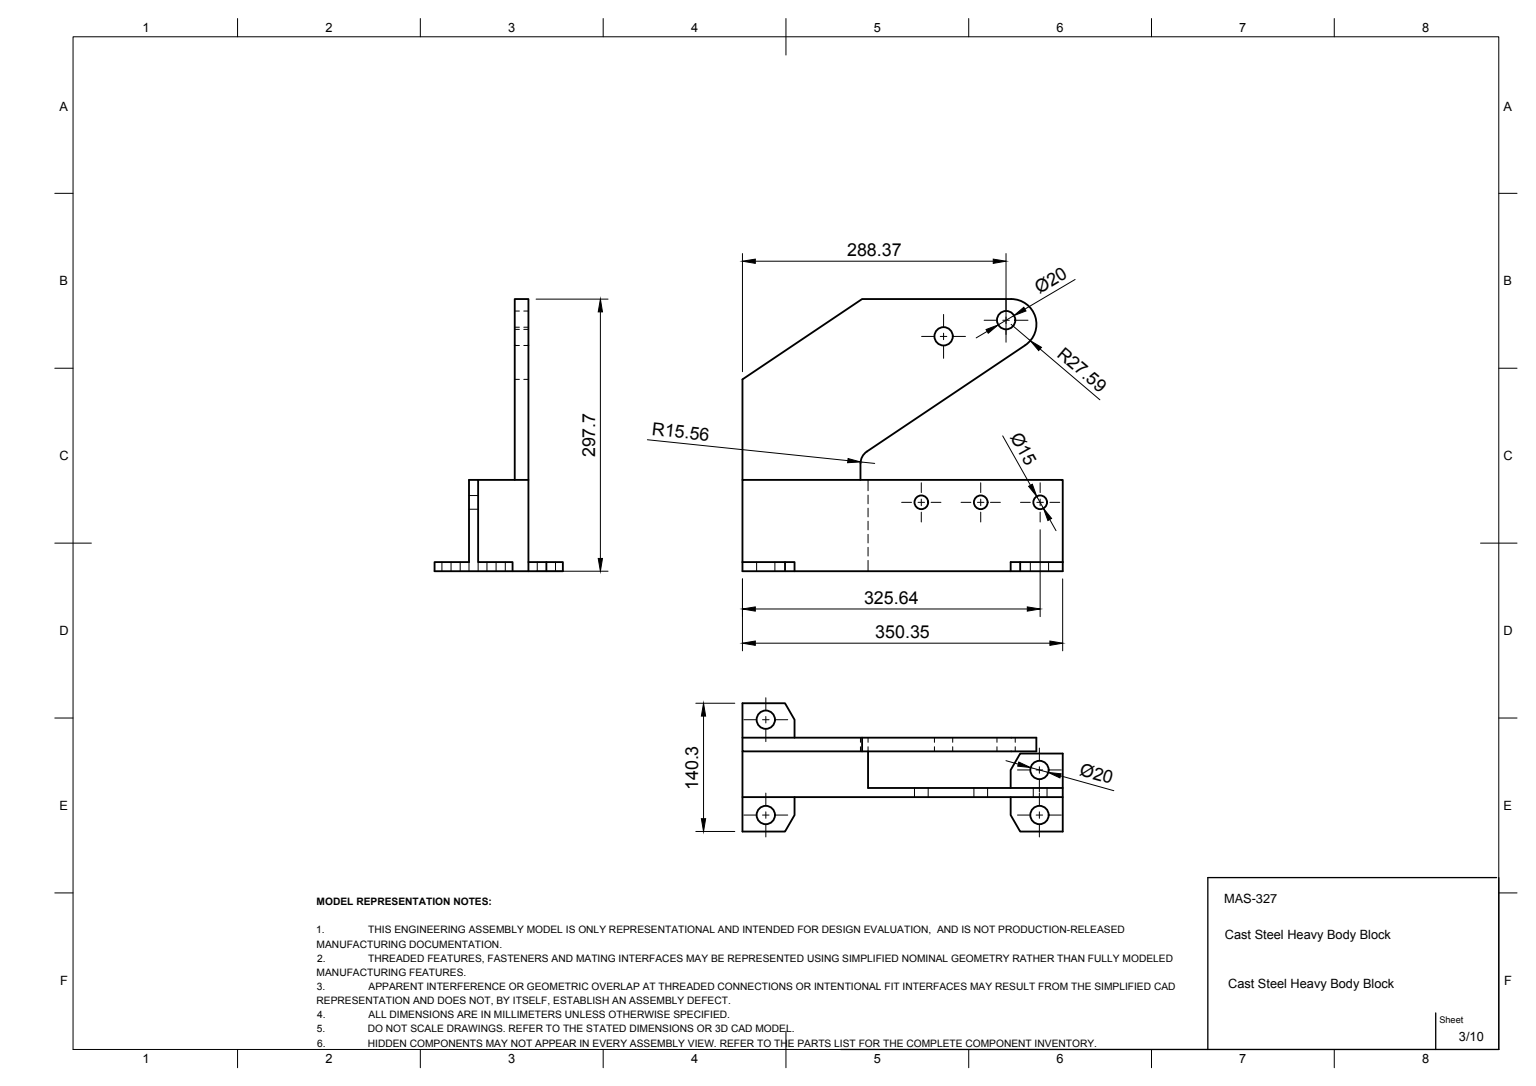
ISO-10303-21;
HEADER;
FILE_DESCRIPTION (('STEP AP214'),
    '1' );
FILE_NAME ('Cast Steel Heavy Body Block.step',
    '2026-10-06T22:16:42',
    ( '' ),
    ( '' ),
    'SwSTEP 2.0',
    'SolidWorks 2025',
    '' );
FILE_SCHEMA (( 'AUTOMOTIVE_DESIGN' ));
ENDSEC;

DATA;
#12=EDGE_LOOP ( 'NONE', ( #7089, #16124, #17025, #12845, #13237 ) ) ;
#25=CIRCLE ( 'NONE', #1445, 7.500000000000007105 ) ;
#26=EDGE_CURVE ( 'NONE', #19406, #2203, #2326, .T. ) ;
#27=ORIENTED_EDGE ( 'NONE', *, *, #7982, .F. ) ;
#40=VERTEX_POINT ( 'NONE', #786 ) ;
#42=ADVANCED_FACE ( 'NONE', ( #9065 ), #564, .F. ) ;
#49=CARTESIAN_POINT ( 'NONE',  ( -120.0322075325610598, -126.9891397928655010, -54.65701158161630246 ) ) ;
#68=VECTOR ( 'NONE', #5817, 1000.000000000000000 ) ;
#70=DIRECTION ( 'NONE',  ( -0.000000000000000000, -0.000000000000000000, 1.000000000000000000 ) ) ;
#85=VECTOR ( 'NONE', #7923, 1000.000000000000000 ) ;
#96=DIRECTION ( 'NONE',  ( -0.000000000000000000, 0.000000000000000000, 1.000000000000000000 ) ) ;
#98=FACE_OUTER_BOUND ( 'NONE', #3212, .T. ) ;
#113=ORIENTED_EDGE ( 'NONE', *, *, #2599, .F. ) ;
#114=CARTESIAN_POINT ( 'NONE',  ( -176.9699209214867324, -136.9891397928655010, -72.64809332337415526 ) ) ;
#119=VERTEX_POINT ( 'NONE', #11350 ) ;
#142=ORIENTED_EDGE ( 'NONE', *, *, #6526, .T. ) ;
#147=EDGE_LOOP ( 'NONE', ( #14360, #18336 ) ) ;
#151=DIRECTION ( 'NONE',  ( 0.000000000000000000, -1.000000000000000000, 0.000000000000000000 ) ) ;
#160=DIRECTION ( 'NONE',  ( -1.000000000000000000, 0.000000000000000000, 0.000000000000000000 ) ) ;
#167=LINE ( 'NONE', #16491, #14475 ) ;
#247=ORIENTED_EDGE ( 'NONE', *, *, #8038, .T. ) ;
#261=VECTOR ( 'NONE', #10869, 1000.000000000000000 ) ;
#269=DIRECTION ( 'NONE',  ( 0.000000000000000000, 0.000000000000000000, 1.000000000000000000 ) ) ;
#270=DIRECTION ( 'NONE',  ( -0.000000000000000000, -0.000000000000000000, -1.000000000000000000 ) ) ;
#278=ORIENTED_EDGE ( 'NONE', *, *, #11475, .T. ) ;
#284=ORIENTED_EDGE ( 'NONE', *, *, #3313, .F. ) ;
#285=VECTOR ( 'NONE', #20979, 1000.000000000000000 ) ;
#315=EDGE_CURVE ( 'NONE', #5215, #4975, #25, .T. ) ;
#328=FACE_OUTER_BOUND ( 'NONE', #18449, .T. ) ;
#380=FACE_OUTER_BOUND ( 'NONE', #4715, .T. ) ;
#417=VERTEX_POINT ( 'NONE', #9257 ) ;
#418=CIRCLE ( 'NONE', #12730, 27.58651506682278765 ) ;
#431=DIRECTION ( 'NONE',  ( 0.000000000000000000, 0.000000000000000000, 1.000000000000000000 ) ) ;
#437=PLANE ( 'NONE',  #12824 ) ;
#465=PLANE ( 'NONE',  #7815 ) ;
#468=ORIENTED_EDGE ( 'NONE', *, *, #12037, .F. ) ;
#478=FACE_OUTER_BOUND ( 'NONE', #9416, .T. ) ;
#509=VECTOR ( 'NONE', #17176, 1000.000000000000000 ) ;
#516=ADVANCED_FACE ( 'NONE', ( #17287, #19278 ), #15850, .F. ) ;
#522=ORIENTED_EDGE ( 'NONE', *, *, #11916, .F. ) ;
#541=CIRCLE ( 'NONE', #5131, 10.00000000000000888 ) ;
#559=FACE_OUTER_BOUND ( 'NONE', #21629, .T. ) ;
#564=CYLINDRICAL_SURFACE ( 'NONE', #18674, 10.00000000000000888 ) ;
#566=ADVANCED_FACE ( 'NONE', ( #7498 ), #12330, .F. ) ;
#590=AXIS2_PLACEMENT_3D ( 'NONE', #17670, #14043, #3917 ) ;
#593=EDGE_CURVE ( 'NONE', #21705, #4967, #4602, .T. ) ;
#601=EDGE_CURVE ( 'NONE', #16938, #20322, #15854, .T. ) ;
#609=LINE ( 'NONE', #7345, #1308 ) ;
#633=CIRCLE ( 'NONE', #13999, 7.500000000000000000 ) ;
#657=DIRECTION ( 'NONE',  ( 0.000000000000000000, 0.000000000000000000, 1.000000000000000000 ) ) ;
#658=ORIENTED_EDGE ( 'NONE', *, *, #12587, .F. ) ;
#668=AXIS2_PLACEMENT_3D ( 'NONE', #14423, #4498, #6045 ) ;
#677=ADVANCED_FACE ( 'NONE', ( #16611 ), #4491, .T. ) ;
#678=CARTESIAN_POINT ( 'NONE',  ( 147.8787791192428074, -126.9891397928655010, 49.65701158161629536 ) ) ;
#682=ORIENTED_EDGE ( 'NONE', *, *, #18825, .F. ) ;
#684=VECTOR ( 'NONE', #722, 1000.000000000000000 ) ;
#706=VERTEX_POINT ( 'NONE', #21264 ) ;
#722=DIRECTION ( 'NONE',  ( 0.000000000000000000, 0.000000000000000000, 1.000000000000000000 ) ) ;
#724=CYLINDRICAL_SURFACE ( 'NONE', #15405, 7.500000000000007105 ) ;
#735=VERTEX_POINT ( 'NONE', #15411 ) ;
#736=VECTOR ( 'NONE', #19488, 1000.000000000000000 ) ;
#761=CARTESIAN_POINT ( 'NONE',  ( 0.000000000000000000, -126.9891397928655010, 0.000000000000000000 ) ) ;
#766=ORIENTED_EDGE ( 'NONE', *, *, #1366, .T. ) ;
#779=DIRECTION ( 'NONE',  ( 0.000000000000000000, 0.000000000000000000, 1.000000000000000000 ) ) ;
#784=VERTEX_POINT ( 'NONE', #6929 ) ;
#786=CARTESIAN_POINT ( 'NONE',  ( -130.4480969619998234, -126.9891397928655010, 67.64809332337415526 ) ) ;
#803=DIRECTION ( 'NONE',  ( 0.000000000000000000, 0.000000000000000000, 1.000000000000000000 ) ) ;
#805=LINE ( 'NONE', #10631, #5353 ) ;
#818=ORIENTED_EDGE ( 'NONE', *, *, #4976, .F. ) ;
#847=ORIENTED_EDGE ( 'NONE', *, *, #6809, .F. ) ;
#850=AXIS2_PLACEMENT_3D ( 'NONE', #17976, #8078, #1233 ) ;
#858=DIRECTION ( 'NONE',  ( 1.000000000000000000, 0.000000000000000000, 5.966140889015784385E-16 ) ) ;
#863=( NAMED_UNIT ( * ) SI_UNIT ( $, .STERADIAN. ) SOLID_ANGLE_UNIT ( ) );
#879=LINE ( 'NONE', #9488, #12922 ) ;
#929=EDGE_CURVE ( 'NONE', #15878, #9201, #3287, .T. ) ;
#943=CYLINDRICAL_SURFACE ( 'NONE', #4707, 10.00000000000000888 ) ;
#965=DIRECTION ( 'NONE',  ( 0.000000000000000000, -1.000000000000000000, 0.000000000000000000 ) ) ;
#970=FILL_AREA_STYLE ('',( #2836 ) ) ;
#1005=DIRECTION ( 'NONE',  ( 0.000000000000000000, 0.000000000000000000, -1.000000000000000000 ) ) ;
#1023=CARTESIAN_POINT ( 'NONE',  ( 116.9721770337685740, 133.1239846058259388, -19.99999999999999289 ) ) ;
#1032=AXIS2_PLACEMENT_3D ( 'NONE', #6238, #19694, #16478 ) ;
#1085=CARTESIAN_POINT ( 'NONE',  ( -120.0322075325610598, -126.9891397928655010, -54.65701158161630246 ) ) ;
#1093=ORIENTED_EDGE ( 'NONE', *, *, #6809, .T. ) ;
#1101=LINE ( 'NONE', #19613, #20236 ) ;
#1116=VERTEX_POINT ( 'NONE', #18932 ) ;
#1131=CARTESIAN_POINT ( 'NONE',  ( -176.9699209214867608, -126.9891397928655010, -35.00000000000000000 ) ) ;
#1139=DIRECTION ( 'NONE',  ( -1.233581138472395521E-15, -0.000000000000000000, 1.000000000000000000 ) ) ;
#1143=ORIENTED_EDGE ( 'NONE', *, *, #9526, .F. ) ;
#1149=DIRECTION ( 'NONE',  ( 0.5010362705417042983, 0.000000000000000000, 0.8654262854811264338 ) ) ;
#1171=ORIENTED_EDGE ( 'NONE', *, *, #13365, .T. ) ;
#1192=DIRECTION ( 'NONE',  ( 1.000000000000000000, 0.000000000000000000, 0.000000000000000000 ) ) ;
#1194=DIRECTION ( 'NONE',  ( 1.000000000000000000, 0.000000000000000000, 0.000000000000000000 ) ) ;
#1208=CARTESIAN_POINT ( 'NONE',  ( -176.9699209214867892, 72.84679049016736485, -25.00000000000000000 ) ) ;
#1224=ORIENTED_EDGE ( 'NONE', *, *, #1690, .F. ) ;
#1225=ORIENTED_EDGE ( 'NONE', *, *, #2133, .T. ) ;
#1233=DIRECTION ( 'NONE',  ( 1.000000000000000000, 0.000000000000000000, 0.000000000000000000 ) ) ;
#1237=CARTESIAN_POINT ( 'NONE',  ( 148.6725454929228079, -61.68114226949890622, 19.99999999999998934 ) ) ;
#1279=ORIENTED_EDGE ( 'NONE', *, *, #10623, .F. ) ;
#1280=ORIENTED_EDGE ( 'NONE', *, *, #9639, .T. ) ;
#1282=EDGE_CURVE ( 'NONE', #4009, #10043, #14611, .T. ) ;
#1302=DIRECTION ( 'NONE',  ( 0.000000000000000000, -1.000000000000000000, 0.000000000000000000 ) ) ;
#1304=CARTESIAN_POINT ( 'NONE',  ( 43.01140435219951996, 119.9070776186055838, -35.00000000000000000 ) ) ;
#1308=VECTOR ( 'NONE', #20782, 1000.000000000000000 ) ;
#1344=DIRECTION ( 'NONE',  ( -0.000000000000000000, 1.000000000000000000, 0.000000000000000000 ) ) ;
#1366=EDGE_CURVE ( 'NONE', #10070, #12769, #541, .T. ) ;
#1408=DIRECTION ( 'NONE',  ( 0.000000000000000000, -1.000000000000000000, 0.000000000000000000 ) ) ;
#1445=AXIS2_PLACEMENT_3D ( 'NONE', #7171, #18740, #10262 ) ;
#1463=ORIENTED_EDGE ( 'NONE', *, *, #1366, .F. ) ;
#1497=CARTESIAN_POINT ( 'NONE',  ( 126.8576204525573274, -136.9891397928655010, 67.64809332337412684 ) ) ;
#1507=FACE_OUTER_BOUND ( 'NONE', #6778, .T. ) ;
#1510=CARTESIAN_POINT ( 'NONE',  ( 116.9721770337685740, 133.1239846058259388, -35.00000000000000000 ) ) ;
#1512=DIRECTION ( 'NONE',  ( 0.000000000000000000, -1.000000000000000000, 0.000000000000000000 ) ) ;
#1527=ORIENTED_EDGE ( 'NONE', *, *, #18029, .T. ) ;
#1535=CARTESIAN_POINT ( 'NONE',  ( -120.0322075325610740, -126.9891397928655010, 49.65701158161630957 ) ) ;
#1538=ADVANCED_FACE ( 'NONE', ( #15287 ), #10546, .F. ) ;
#1542=CARTESIAN_POINT ( 'NONE',  ( -151.4692556286852891, -126.9891397928655010, -64.65701158161634510 ) ) ;
#1543=EDGE_CURVE ( 'NONE', #18069, #12813, #20253, .T. ) ;
#1569=DIRECTION ( 'NONE',  ( -1.000000000000000000, 0.000000000000000000, 0.000000000000000000 ) ) ;
#1573=VERTEX_POINT ( 'NONE', #18482 ) ;
#1581=AXIS2_PLACEMENT_3D ( 'NONE', #1237, #19759, #16328 ) ;
#1601=AXIS2_PLACEMENT_3D ( 'NONE', #19582, #1512, #8350 ) ;
#1608=VERTEX_POINT ( 'NONE', #16926 ) ;
#1612=CYLINDRICAL_SURFACE ( 'NONE', #21460, 7.500000000000007105 ) ;
#1631=DIRECTION ( 'NONE',  ( 0.000000000000000000, -1.000000000000000000, 0.000000000000000000 ) ) ;
#1635=DIRECTION ( 'NONE',  ( 1.000000000000000000, 0.000000000000000000, 0.000000000000000000 ) ) ;
#1636=EDGE_LOOP ( 'NONE', ( #13666, #2702 ) ) ;
#1646=LINE ( 'NONE', #11664, #7653 ) ;
#1662=EDGE_CURVE ( 'NONE', #9722, #11465, #14251, .T. ) ;
#1665=EDGE_LOOP ( 'NONE', ( #5611, #19532, #4554, #12412 ) ) ;
#1668=EDGE_CURVE ( 'NONE', #4967, #19403, #16139, .T. ) ;
#1680=CARTESIAN_POINT ( 'NONE',  ( 18.67254549292281141, -61.68114226949890622, 30.00000000000000000 ) ) ;
#1690=EDGE_CURVE ( 'NONE', #12769, #10070, #4754, .T. ) ;
#1692=CARTESIAN_POINT ( 'NONE',  ( -39.63192160874135084, -37.13255853780189852, 20.00000000000002132 ) ) ;
#1696=VERTEX_POINT ( 'NONE', #5891 ) ;
#1702=DIRECTION ( 'NONE',  ( 0.000000000000000000, -1.000000000000000000, 0.000000000000000000 ) ) ;
#1707=DIRECTION ( 'NONE',  ( 0.000000000000000000, -1.000000000000000000, 0.000000000000000000 ) ) ;
#1709=CARTESIAN_POINT ( 'NONE',  ( -151.4692556286852891, -136.9891397928655010, 39.65701158161630246 ) ) ;
#1729=CARTESIAN_POINT ( 'NONE',  ( 173.3794444120442506, -126.9891397928655010, 67.64809332337412684 ) ) ;
#1741=DIRECTION ( 'NONE',  ( -0.000000000000000000, -0.000000000000000000, 1.000000000000000000 ) ) ;
#1760=CARTESIAN_POINT ( 'NONE',  ( -176.9699209214867608, -136.9891397928655010, -35.00000000000000000 ) ) ;
#1768=DIRECTION ( 'NONE',  ( 1.000000000000000000, 0.000000000000000000, 5.966140889015784385E-16 ) ) ;
#1773=EDGE_CURVE ( 'NONE', #11679, #1573, #7680, .T. ) ;
#1794=AXIS2_PLACEMENT_3D ( 'NONE', #761, #5605, #2201 ) ;
#1804=ORIENTED_EDGE ( 'NONE', *, *, #20245, .T. ) ;
#1807=ORIENTED_EDGE ( 'NONE', *, *, #15853, .T. ) ;
#1836=VECTOR ( 'NONE', #5777, 1000.000000000000000 ) ;
#1840=CARTESIAN_POINT ( 'NONE',  ( 26.17254549292281141, -61.68114226949890622, 30.00000000000000000 ) ) ;
#1856=CARTESIAN_POINT ( 'NONE',  ( 116.9721770337685740, 133.1239846058259388, -19.99999999999999289 ) ) ;
#1866=CARTESIAN_POINT ( 'NONE',  ( -40.97538603781489996, -6.141859983696325465, -25.00000000000000000 ) ) ;
#1898=AXIS2_PLACEMENT_3D ( 'NONE', #17581, #5791, #9447 ) ;
#1899=ORIENTED_EDGE ( 'NONE', *, *, #8843, .F. ) ;
#1913=CYLINDRICAL_SURFACE ( 'NONE', #20496, 10.00000000000003730 ) ;
#1934=EDGE_CURVE ( 'NONE', #21705, #12683, #2918, .T. ) ;
#1936=EDGE_LOOP ( 'NONE', ( #10832, #15493, #3293, #10748, #3973, #12663, #1527, #9500 ) ) ;
#1979=VECTOR ( 'NONE', #8089, 1000.000000000000000 ) ;
#1997=VECTOR ( 'NONE', #12476, 1000.000000000000000 ) ;
#2032=CYLINDRICAL_SURFACE ( 'NONE', #3445, 27.58651506682278765 ) ;
#2041=CARTESIAN_POINT ( 'NONE',  ( 126.8576204525573274, -136.9891397928655010, -17.64809332337413750 ) ) ;
#2042=CARTESIAN_POINT ( 'NONE',  ( -88.69383338279318707, 132.1114735047150646, -19.99999999999996803 ) ) ;
#2046=AXIS2_PLACEMENT_3D ( 'NONE', #16795, #15260, #13597 ) ;
#2082=DIRECTION ( 'NONE',  ( -1.000000000000000000, 0.000000000000000000, -0.000000000000000000 ) ) ;
#2089=DIRECTION ( 'NONE',  ( 1.186952418100008983E-16, 0.000000000000000000, 1.000000000000000000 ) ) ;
#2092=CARTESIAN_POINT ( 'NONE',  ( 173.3794444120442222, -354.7018910364275257, 19.99999999999999645 ) ) ;
#2095=EDGE_LOOP ( 'NONE', ( #16991, #14494, #15108, #12297 ) ) ;
#2133=EDGE_CURVE ( 'NONE', #3147, #7116, #5434, .T. ) ;
#2143=DIRECTION ( 'NONE',  ( 0.000000000000000000, -1.000000000000000000, 0.000000000000000000 ) ) ;
#2145=ORIENTED_EDGE ( 'NONE', *, *, #9831, .T. ) ;
#2157=CARTESIAN_POINT ( 'NONE',  ( 26.17254549292281141, -61.68114226949890622, -46.21320343559645494 ) ) ;
#2160=CARTESIAN_POINT ( 'NONE',  ( 101.4021762516569822, 137.5714195593754710, -35.00000000000000000 ) ) ;
#2161=CARTESIAN_POINT ( 'NONE',  ( 53.01140435219953417, 119.9070776186055838, -35.00000000000000000 ) ) ;
#2175=ORIENTED_EDGE ( 'NONE', *, *, #7095, .T. ) ;
#2177=CARTESIAN_POINT ( 'NONE',  ( -151.4692556286852891, -126.9891397928655010, 39.65701158161630246 ) ) ;
#2188=AXIS2_PLACEMENT_3D ( 'NONE', #13387, #4899, #6555 ) ;
#2201=DIRECTION ( 'NONE',  ( 0.000000000000000000, -0.000000000000000000, -1.000000000000000000 ) ) ;
#2203=VERTEX_POINT ( 'NONE', #3476 ) ;
#2258=CARTESIAN_POINT ( 'NONE',  ( -151.4692556286852891, -136.9891397928655010, 59.65701158161632378 ) ) ;
#2276=EDGE_CURVE ( 'NONE', #17291, #7232, #14977, .T. ) ;
#2280=DIRECTION ( 'NONE',  ( 1.000000000000000000, 0.000000000000000000, 0.000000000000000000 ) ) ;
#2294=CARTESIAN_POINT ( 'NONE',  ( 144.5586921005913439, 482.8605407899846682, -19.99999999999999645 ) ) ;
#2326=LINE ( 'NONE', #2647, #3184 ) ;
#2328=ADVANCED_FACE ( 'NONE', ( #4870, #11807 ), #14783, .T. ) ;
#2331=ORIENTED_EDGE ( 'NONE', *, *, #10158, .F. ) ;
#2334=CIRCLE ( 'NONE', #19236, 10.00000000000003730 ) ;
#2344=VECTOR ( 'NONE', #431, 1000.000000000000000 ) ;
#2377=ADVANCED_FACE ( 'NONE', ( #13468 ), #13138, .F. ) ;
#2403=CARTESIAN_POINT ( 'NONE',  ( 0.000000000000000000, 0.000000000000000000, 0.000000000000000000 ) ) ;
#2404=DIRECTION ( 'NONE',  ( -0.000000000000000000, -0.000000000000000000, 1.000000000000000000 ) ) ;
#2405=DIRECTION ( 'NONE',  ( 0.000000000000000000, 0.000000000000000000, -1.000000000000000000 ) ) ;
#2456=ORIENTED_EDGE ( 'NONE', *, *, #8916, .F. ) ;
#2466=ORIENTED_EDGE ( 'NONE', *, *, #13663, .T. ) ;
#2479=DIRECTION ( 'NONE',  ( -0.000000000000000000, -0.000000000000000000, 1.000000000000000000 ) ) ;
#2496=DIRECTION ( 'NONE',  ( -0.000000000000000000, -0.000000000000000000, 1.000000000000000000 ) ) ;
#2507=LINE ( 'NONE', #19268, #16704 ) ;
#2512=SURFACE_STYLE_FILL_AREA ( #970 ) ;
#2527=AXIS2_PLACEMENT_3D ( 'NONE', #10957, #17666, #9308 ) ;
#2536=CARTESIAN_POINT ( 'NONE',  ( -176.9699209214867892, 72.84679049016739327, -19.99999999999995737 ) ) ;
#2549=EDGE_CURVE ( 'NONE', #15790, #784, #8294, .T. ) ;
#2562=DIRECTION ( 'NONE',  ( -0.000000000000000000, -0.000000000000000000, -1.000000000000000000 ) ) ;
#2563=EDGE_LOOP ( 'NONE', ( #11816, #5747, #14579, #3772 ) ) ;
#2574=VERTEX_POINT ( 'NONE', #13676 ) ;
#2580=CARTESIAN_POINT ( 'NONE',  ( 173.3794444120442506, -136.9891397928655010, -17.64809332337413750 ) ) ;
#2599=EDGE_CURVE ( 'NONE', #3989, #14342, #7299, .T. ) ;
#2611=DIRECTION ( 'NONE',  ( 1.000000000000000000, 0.000000000000000000, 0.000000000000000000 ) ) ;
#2616=SURFACE_SIDE_STYLE ('',( #2512 ) ) ;
#2625=DIRECTION ( 'NONE',  ( 0.000000000000000000, -1.000000000000000000, 0.000000000000000000 ) ) ;
#2637=LINE ( 'NONE', #1208, #3416 ) ;
#2639=DIRECTION ( 'NONE',  ( 0.000000000000000000, 0.000000000000000000, -1.000000000000000000 ) ) ;
#2647=CARTESIAN_POINT ( 'NONE',  ( 144.5586921005913439, 133.1239846058259388, -25.00000000000000000 ) ) ;
#2663=UNCERTAINTY_MEASURE_WITH_UNIT (LENGTH_MEASURE( 1.000000000000000082E-05 ), #12101, 'distance_accuracy_value', 'NONE');
#2673=EDGE_LOOP ( 'NONE', ( #7016, #20805 ) ) ;
#2675=CIRCLE ( 'NONE', #7981, 10.00000000000000888 ) ;
#2702=ORIENTED_EDGE ( 'NONE', *, *, #5054, .F. ) ;
#2719=CARTESIAN_POINT ( 'NONE',  ( 116.9721770337685882, 160.7104996726487514, -35.00000000000000000 ) ) ;
#2737=CARTESIAN_POINT ( 'NONE',  ( -47.86331837773882825, -37.13255853780189852, -25.00000000000000000 ) ) ;
#2740=VECTOR ( 'NONE', #14647, 1000.000000000000000 ) ;
#2742=VERTEX_POINT ( 'NONE', #3765 ) ;
#2748=CARTESIAN_POINT ( 'NONE',  ( 26.17254549292281141, -61.68114226949890622, 20.00000000000000355 ) ) ;
#2774=ADVANCED_FACE ( 'NONE', ( #4505 ), #14211, .F. ) ;
#2782=ORIENTED_EDGE ( 'NONE', *, *, #11167, .F. ) ;
#2798=EDGE_CURVE ( 'NONE', #12363, #19770, #19292, .T. ) ;
#2800=VECTOR ( 'NONE', #6103, 1000.000000000000000 ) ;
#2814=LINE ( 'NONE', #14493, #10358 ) ;
#2836=FILL_AREA_STYLE_COLOUR ( '', #20940 ) ;
#2837=CARTESIAN_POINT ( 'NONE',  ( -120.0322075325610740, -126.9891397928655010, 49.65701158161630957 ) ) ;
#2838=CARTESIAN_POINT ( 'NONE',  ( 173.3794444120442506, -126.9891397928655010, 19.99999999999999645 ) ) ;
#2839=LINE ( 'NONE', #9580, #85 ) ;
#2841=CARTESIAN_POINT ( 'NONE',  ( 116.9721770337685740, 133.1239846058259388, -25.00000000000000000 ) ) ;
#2853=DIRECTION ( 'NONE',  ( -0.000000000000000000, -0.000000000000000000, 1.000000000000000000 ) ) ;
#2856=DIRECTION ( 'NONE',  ( 1.000000000000000000, -0.000000000000000000, -0.000000000000000000 ) ) ;
#2872=ORIENTED_EDGE ( 'NONE', *, *, #5164, .F. ) ;
#2873=ORIENTED_EDGE ( 'NONE', *, *, #19692, .F. ) ;
#2880=CIRCLE ( 'NONE', #15211, 10.00000000000000888 ) ;
#2918=LINE ( 'NONE', #6560, #10778 ) ;
#2932=EDGE_LOOP ( 'NONE', ( #3098, #5240 ) ) ;
#2954=LINE ( 'NONE', #10911, #8544 ) ;
#2957=DIRECTION ( 'NONE',  ( 0.000000000000000000, -1.000000000000000000, 0.000000000000000000 ) ) ;
#2958=ADVANCED_FACE ( 'NONE', ( #16298 ), #19724, .T. ) ;
#2967=ADVANCED_BREP_SHAPE_REPRESENTATION ( '', ( #7648, #12657 ), #7388 ) ;
#2984=ORIENTED_EDGE ( 'NONE', *, *, #11356, .F. ) ;
#2994=VECTOR ( 'NONE', #5145, 1000.000000000000000 ) ;
#3009=ORIENTED_EDGE ( 'NONE', *, *, #8423, .F. ) ;
#3014=AXIS2_PLACEMENT_3D ( 'NONE', #17733, #19730, #2639 ) ;
#3015=EDGE_LOOP ( 'NONE', ( #12043, #12503, #17690, #7873 ) ) ;
#3022=CARTESIAN_POINT ( 'NONE',  ( -176.9699209214867892, -37.13255853780189852, 30.00000000000000000 ) ) ;
#3035=ORIENTED_EDGE ( 'NONE', *, *, #11167, .T. ) ;
#3041=EDGE_LOOP ( 'NONE', ( #18081, #20830, #4851, #15021 ) ) ;
#3043=AXIS2_PLACEMENT_3D ( 'NONE', #14344, #7530, #10618 ) ;
#3059=FACE_OUTER_BOUND ( 'NONE', #1936, .T. ) ;
#3079=DIRECTION ( 'NONE',  ( 5.966140889015784385E-16, 0.000000000000000000, -1.000000000000000000 ) ) ;
#3081=CARTESIAN_POINT ( 'NONE',  ( 11.17254549292281318, -61.68114226949890622, 20.00000000000000355 ) ) ;
#3084=CARTESIAN_POINT ( 'NONE',  ( 83.67254549292280785, -61.68114226949890622, 20.00000000000000355 ) ) ;
#3098=ORIENTED_EDGE ( 'NONE', *, *, #12468, .F. ) ;
#3099=ORIENTED_EDGE ( 'NONE', *, *, #7039, .F. ) ;
#3110=DIRECTION ( 'NONE',  ( 0.000000000000000000, -1.000000000000000000, 0.000000000000000000 ) ) ;
#3113=CARTESIAN_POINT ( 'NONE',  ( 141.1725454929228079, -61.68114226949890622, 30.00000000000000000 ) ) ;
#3147=VERTEX_POINT ( 'NONE', #19051 ) ;
#3159=EDGE_CURVE ( 'NONE', #2574, #14607, #20383, .T. ) ;
#3179=ORIENTED_EDGE ( 'NONE', *, *, #26, .F. ) ;
#3183=CARTESIAN_POINT ( 'NONE',  ( 147.8787791192428074, -136.9891397928655010, 10.34298841838370642 ) ) ;
#3184=VECTOR ( 'NONE', #9389, 1000.000000000000000 ) ;
#3193=FACE_OUTER_BOUND ( 'NONE', #7898, .T. ) ;
#3212=EDGE_LOOP ( 'NONE', ( #10152, #12911, #16288, #16341 ) ) ;
#3240=ORIENTED_EDGE ( 'NONE', *, *, #16105, .T. ) ;
#3275=DIRECTION ( 'NONE',  ( -1.000000000000000000, 0.000000000000000000, -2.437363037925170562E-16 ) ) ;
#3276=EDGE_CURVE ( 'NONE', #8458, #14342, #14465, .T. ) ;
#3280=LINE ( 'NONE', #12898, #5354 ) ;
#3282=CARTESIAN_POINT ( 'NONE',  ( 0.000000000000000000, -37.13255853780189852, 30.00000000000000000 ) ) ;
#3287=LINE ( 'NONE', #16720, #10407 ) ;
#3291=CIRCLE ( 'NONE', #15601, 10.00000000000003730 ) ;
#3293=ORIENTED_EDGE ( 'NONE', *, *, #3630, .T. ) ;
#3313=EDGE_CURVE ( 'NONE', #15277, #4525, #17769, .T. ) ;
#3321=ORIENTED_EDGE ( 'NONE', *, *, #8843, .T. ) ;
#3323=ORIENTED_EDGE ( 'NONE', *, *, #1773, .F. ) ;
#3329=CARTESIAN_POINT ( 'NONE',  ( 0.000000000000000000, -126.9891397928655010, 0.000000000000000000 ) ) ;
#3332=FACE_OUTER_BOUND ( 'NONE', #19635, .T. ) ;
#3337=ORIENTED_EDGE ( 'NONE', *, *, #6526, .F. ) ;
#3353=CARTESIAN_POINT ( 'NONE',  ( -151.4692556286852891, -136.9891397928655010, -54.65701158161630246 ) ) ;
#3363=DIRECTION ( 'NONE',  ( 1.000000000000000000, 0.000000000000000000, 0.000000000000000000 ) ) ;
#3378=ORIENTED_EDGE ( 'NONE', *, *, #4559, .T. ) ;
#3391=EDGE_CURVE ( 'NONE', #13430, #16995, #21315, .T. ) ;
#3396=DIRECTION ( 'NONE',  ( -0.5010362705417047424, 0.000000000000000000, -0.8654262854811261008 ) ) ;
#3408=EDGE_LOOP ( 'NONE', ( #14606, #4517, #12471, #2782 ) ) ;
#3416=VECTOR ( 'NONE', #779, 1000.000000000000000 ) ;
#3436=VECTOR ( 'NONE', #13943, 1000.000000000000000 ) ;
#3445=AXIS2_PLACEMENT_3D ( 'NONE', #18461, #269, #3363 ) ;
#3476=CARTESIAN_POINT ( 'NONE',  ( 144.5586921005913439, 133.1239846058259388, -19.99999999999999645 ) ) ;
#3485=ORIENTED_EDGE ( 'NONE', *, *, #21498, .T. ) ;
#3495=FACE_OUTER_BOUND ( 'NONE', #12, .T. ) ;
#3508=CARTESIAN_POINT ( 'NONE',  ( 147.8787791192428074, -126.9891397928655010, 10.34298841838370642 ) ) ;
#3564=EDGE_CURVE ( 'NONE', #1573, #10861, #4803, .T. ) ;
#3569=ORIENTED_EDGE ( 'NONE', *, *, #6191, .F. ) ;
#3577=FACE_OUTER_BOUND ( 'NONE', #19092, .T. ) ;
#3598=CIRCLE ( 'NONE', #12744, 10.00000000000003730 ) ;
#3630=EDGE_CURVE ( 'NONE', #12363, #20108, #7922, .T. ) ;
#3648=FACE_OUTER_BOUND ( 'NONE', #12386, .T. ) ;
#3667=EDGE_LOOP ( 'NONE', ( #7526, #9262, #18046, #20185, #3337, #5414, #10888, #19284, #4437, #9397, #14577, #6175, #1280 ) ) ;
#3674=ORIENTED_EDGE ( 'NONE', *, *, #13573, .T. ) ;
#3677=CARTESIAN_POINT ( 'NONE',  ( -151.4692556286852891, -136.9891397928655010, -64.65701158161634510 ) ) ;
#3684=EDGE_CURVE ( 'NONE', #9201, #4525, #14843, .T. ) ;
#3687=FACE_OUTER_BOUND ( 'NONE', #19743, .T. ) ;
#3730=DIRECTION ( 'NONE',  ( 1.000000000000000000, 0.000000000000000000, -1.257660470541341077E-16 ) ) ;
#3755=DIRECTION ( 'NONE',  ( 1.000000000000000000, 0.000000000000000000, -0.000000000000000000 ) ) ;
#3758=AXIS2_PLACEMENT_3D ( 'NONE', #6028, #965, #2405 ) ;
#3765=CARTESIAN_POINT ( 'NONE',  ( 91.17254549292282206, -61.68114226949890622, 20.00000000000000355 ) ) ;
#3772=ORIENTED_EDGE ( 'NONE', *, *, #2599, .T. ) ;
#3786=CARTESIAN_POINT ( 'NONE',  ( 126.8576204525573274, -126.9891397928655010, -17.64809332337413750 ) ) ;
#3789=AXIS2_PLACEMENT_3D ( 'NONE', #3084, #18514, #10036 ) ;
#3796=CARTESIAN_POINT ( 'NONE',  ( 156.1725454929228079, -61.68114226949890622, 30.00000000000000000 ) ) ;
#3805=VECTOR ( 'NONE', #20027, 1000.000000000000000 ) ;
#3833=ADVANCED_FACE ( 'NONE', ( #16828 ), #15183, .F. ) ;
#3873=DIRECTION ( 'NONE',  ( -0.000000000000000000, -0.000000000000000000, -1.000000000000000000 ) ) ;
#3883=ORIENTED_EDGE ( 'NONE', *, *, #18144, .F. ) ;
#3903=ADVANCED_FACE ( 'NONE', ( #13739 ), #8684, .T. ) ;
#3917=DIRECTION ( 'NONE',  ( 0.000000000000000000, 0.000000000000000000, -1.000000000000000000 ) ) ;
#3920=CARTESIAN_POINT ( 'NONE',  ( 18.67254549292281141, -61.68114226949890622, -46.21320343559645494 ) ) ;
#3953=( NAMED_UNIT ( * ) PLANE_ANGLE_UNIT ( ) SI_UNIT ( $, .RADIAN. ) );
#3973=ORIENTED_EDGE ( 'NONE', *, *, #14257, .F. ) ;
#3983=DIRECTION ( 'NONE',  ( 0.000000000000000000, 0.000000000000000000, 1.000000000000000000 ) ) ;
#3989=VERTEX_POINT ( 'NONE', #11873 ) ;
#4009=VERTEX_POINT ( 'NONE', #3508 ) ;
#4021=CARTESIAN_POINT ( 'NONE',  ( 126.8576204525573274, -136.9891397928655010, 67.64809332337412684 ) ) ;
#4026=DIRECTION ( 'NONE',  ( 0.000000000000000000, 0.000000000000000000, -1.000000000000000000 ) ) ;
#4035=LINE ( 'NONE', #17574, #9321 ) ;
#4051=DIRECTION ( 'NONE',  ( 0.8302490056034136368, 0.5573926701119623628, 0.000000000000000000 ) ) ;
#4082=LINE ( 'NONE', #16079, #10825 ) ;
#4084=CARTESIAN_POINT ( 'NONE',  ( 116.4417310231185780, -136.9891397928655010, 30.00000000000000000 ) ) ;
#4086=CARTESIAN_POINT ( 'NONE',  ( 147.8787791192428074, -126.9891397928655010, -9.657011581616311346 ) ) ;
#4091=ORIENTED_EDGE ( 'NONE', *, *, #9801, .T. ) ;
#4104=LINE ( 'NONE', #12590, #16410 ) ;
#4110=AXIS2_PLACEMENT_3D ( 'NONE', #21112, #19234, #13938 ) ;
#4113=DIRECTION ( 'NONE',  ( 0.000000000000000000, -1.000000000000000000, 0.000000000000000000 ) ) ;
#4134=DIRECTION ( 'NONE',  ( 0.000000000000000000, 0.000000000000000000, 1.000000000000000000 ) ) ;
#4138=CARTESIAN_POINT ( 'NONE',  ( -176.9699209214867608, -126.9891397928655010, -35.00000000000000000 ) ) ;
#4145=CARTESIAN_POINT ( 'NONE',  ( 116.4417310231185780, -126.9891397928655010, 49.65701158161629536 ) ) ;
#4198=DIRECTION ( 'NONE',  ( -0.000000000000000000, -0.000000000000000000, 1.000000000000000000 ) ) ;
#4199=ORIENTED_EDGE ( 'NONE', *, *, #8423, .T. ) ;
#4205=ORIENTED_EDGE ( 'NONE', *, *, #14991, .T. ) ;
#4218=DIRECTION ( 'NONE',  ( 0.000000000000000000, -1.000000000000000000, 0.000000000000000000 ) ) ;
#4238=DIRECTION ( 'NONE',  ( -1.000000000000000000, -0.000000000000000000, -0.000000000000000000 ) ) ;
#4244=EDGE_CURVE ( 'NONE', #14342, #3147, #17903, .T. ) ;
#4268=FACE_OUTER_BOUND ( 'NONE', #3015, .T. ) ;
#4279=LINE ( 'NONE', #4605, #7485 ) ;
#4283=ADVANCED_FACE ( 'NONE', ( #16257, #8227, #6228, #19564 ), #18247, .F. ) ;
#4286=AXIS2_PLACEMENT_3D ( 'NONE', #11428, #15955, #4377 ) ;
#4299=ORIENTED_EDGE ( 'NONE', *, *, #12587, .T. ) ;
#4318=CARTESIAN_POINT ( 'NONE',  ( -120.0322075325610740, -126.9891397928655010, 49.65701158161630957 ) ) ;
#4320=CARTESIAN_POINT ( 'NONE',  ( 173.3794444120442506, -126.9891397928655010, -17.64809332337413750 ) ) ;
#4343=DIRECTION ( 'NONE',  ( -1.140132994654635861E-16, -0.000000000000000000, -1.000000000000000000 ) ) ;
#4357=ORIENTED_EDGE ( 'NONE', *, *, #2133, .F. ) ;
#4369=CARTESIAN_POINT ( 'NONE',  ( -47.86331837773882825, -19.06233958201669765, -19.99999999999997513 ) ) ;
#4377=DIRECTION ( 'NONE',  ( 0.000000000000000000, 0.000000000000000000, 1.000000000000000000 ) ) ;
#4406=EDGE_LOOP ( 'NONE', ( #468, #5418 ) ) ;
#4417=AXIS2_PLACEMENT_3D ( 'NONE', #3329, #1344, #4753 ) ;
#4437=ORIENTED_EDGE ( 'NONE', *, *, #18399, .F. ) ;
#4446=DIRECTION ( 'NONE',  ( -1.140132994654635861E-16, -0.000000000000000000, -1.000000000000000000 ) ) ;
#4447=CARTESIAN_POINT ( 'NONE',  ( -46.09493621325655255, 160.7104996726487514, -35.00000000000000000 ) ) ;
#4457=CARTESIAN_POINT ( 'NONE',  ( 147.8787791192428074, -126.9891397928655010, 49.65701158161629536 ) ) ;
#4461=VECTOR ( 'NONE', #11444, 1000.000000000000000 ) ;
#4478=DIRECTION ( 'NONE',  ( 0.000000000000000000, 0.000000000000000000, 1.000000000000000000 ) ) ;
#4486=DIRECTION ( 'NONE',  ( 0.5010362705417046314, -0.000000000000000000, -0.8654262854811262118 ) ) ;
#4491=CYLINDRICAL_SURFACE ( 'NONE', #20957, 27.58651506682278765 ) ;
#4493=ORIENTED_EDGE ( 'NONE', *, *, #11250, .T. ) ;
#4498=DIRECTION ( 'NONE',  ( 0.000000000000000000, -1.000000000000000000, 0.000000000000000000 ) ) ;
#4505=FACE_OUTER_BOUND ( 'NONE', #6908, .T. ) ;
#4513=DIRECTION ( 'NONE',  ( 0.000000000000000000, -1.000000000000000000, 0.000000000000000000 ) ) ;
#4517=ORIENTED_EDGE ( 'NONE', *, *, #10557, .T. ) ;
#4524=EDGE_LOOP ( 'NONE', ( #21426, #12231, #11115, #17402 ) ) ;
#4525=VERTEX_POINT ( 'NONE', #2041 ) ;
#4528=ORIENTED_EDGE ( 'NONE', *, *, #16312, .T. ) ;
#4541=ORIENTED_EDGE ( 'NONE', *, *, #9639, .F. ) ;
#4547=ORIENTED_EDGE ( 'NONE', *, *, #3159, .T. ) ;
#4549=AXIS2_PLACEMENT_3D ( 'NONE', #1856, #11988, #3730 ) ;
#4552=VERTEX_POINT ( 'NONE', #10211 ) ;
#4554=ORIENTED_EDGE ( 'NONE', *, *, #18688, .T. ) ;
#4559=EDGE_CURVE ( 'NONE', #2742, #10861, #10424, .T. ) ;
#4560=VECTOR ( 'NONE', #5254, 1000.000000000000000 ) ;
#4573=VERTEX_POINT ( 'NONE', #6573 ) ;
#4600=FACE_OUTER_BOUND ( 'NONE', #20484, .T. ) ;
#4602=LINE ( 'NONE', #2737, #736 ) ;
#4605=CARTESIAN_POINT ( 'NONE',  ( 147.8787791192428074, -126.9891397928655010, 10.34298841838370642 ) ) ;
#4616=DIRECTION ( 'NONE',  ( -0.000000000000000000, 0.000000000000000000, 1.000000000000000000 ) ) ;
#4624=PLANE ( 'NONE',  #20503 ) ;
#4636=AXIS2_PLACEMENT_3D ( 'NONE', #12352, #4198, #18976 ) ;
#4667=ORIENTED_EDGE ( 'NONE', *, *, #7095, .F. ) ;
#4674=CARTESIAN_POINT ( 'NONE',  ( -47.86331837773882825, -37.13255853780189852, -35.00000000000000000 ) ) ;
#4676=CARTESIAN_POINT ( 'NONE',  ( -176.9699209214867608, -126.9891397928655010, 67.64809332337415526 ) ) ;
#4679=SHAPE_DEFINITION_REPRESENTATION ( #16619, #5457 ) ;
#4685=LINE ( 'NONE', #11401, #6629 ) ;
#4707=AXIS2_PLACEMENT_3D ( 'NONE', #4457, #21235, #10880 ) ;
#4713=ORIENTED_EDGE ( 'NONE', *, *, #19345, .F. ) ;
#4715=EDGE_LOOP ( 'NONE', ( #13255, #818, #19200, #6200 ) ) ;
#4745=VERTEX_POINT ( 'NONE', #7338 ) ;
#4753=DIRECTION ( 'NONE',  ( 0.000000000000000000, -0.000000000000000000, 1.000000000000000000 ) ) ;
#4754=CIRCLE ( 'NONE', #17070, 10.00000000000000888 ) ;
#4755=CARTESIAN_POINT ( 'NONE',  ( -176.9699209214867608, -136.9891397928655010, 67.64809332337415526 ) ) ;
#4756=CARTESIAN_POINT ( 'NONE',  ( -130.4480969619997950, -126.9891397928655010, -72.64809332337412684 ) ) ;
#4781=LINE ( 'NONE', #9758, #9063 ) ;
#4800=EDGE_LOOP ( 'NONE', ( #6765, #7173, #12032, #19175, #16521 ) ) ;
#4803=CIRCLE ( 'NONE', #5853, 7.500000000000007105 ) ;
#4843=LINE ( 'NONE', #8160, #13614 ) ;
#4851=ORIENTED_EDGE ( 'NONE', *, *, #5054, .T. ) ;
#4859=VERTEX_POINT ( 'NONE', #8327 ) ;
#4870=FACE_BOUND ( 'NONE', #2673, .T. ) ;
#4874=ADVANCED_FACE ( 'NONE', ( #18571 ), #2032, .T. ) ;
#4877=VERTEX_POINT ( 'NONE', #1709 ) ;
#4884=CARTESIAN_POINT ( 'NONE',  ( -47.86331837773882825, -19.06233958201669765, -25.00000000000000000 ) ) ;
#4899=DIRECTION ( 'NONE',  ( 0.8654262854811263228, 0.000000000000000000, 0.5010362705417044094 ) ) ;
#4906=VECTOR ( 'NONE', #16157, 1000.000000000000000 ) ;
#4911=ADVANCED_FACE ( 'NONE', ( #3687 ), #8654, .T. ) ;
#4925=ADVANCED_FACE ( 'NONE', ( #380 ), #7109, .T. ) ;
#4947=ORIENTED_EDGE ( 'NONE', *, *, #12147, .T. ) ;
#4960=CARTESIAN_POINT ( 'NONE',  ( 101.4021762516569822, 137.5714195593754710, -19.99999999999997868 ) ) ;
#4967=VERTEX_POINT ( 'NONE', #13917 ) ;
#4975=VERTEX_POINT ( 'NONE', #3796 ) ;
#4976=EDGE_CURVE ( 'NONE', #4552, #18638, #19112, .T. ) ;
#5004=EDGE_LOOP ( 'NONE', ( #8112, #1224, #12965, #21215 ) ) ;
#5006=EDGE_LOOP ( 'NONE', ( #4357, #10188, #7668, #4493 ) ) ;
#5014=DIRECTION ( 'NONE',  ( -0.000000000000000000, -0.000000000000000000, 1.000000000000000000 ) ) ;
#5026=ORIENTED_EDGE ( 'NONE', *, *, #6493, .F. ) ;
#5054=EDGE_CURVE ( 'NONE', #10397, #4877, #9074, .T. ) ;
#5055=EDGE_LOOP ( 'NONE', ( #522, #9829 ) ) ;
#5077=ORIENTED_EDGE ( 'NONE', *, *, #5202, .F. ) ;
#5123=CARTESIAN_POINT ( 'NONE',  ( 116.4417310231185780, -136.9891397928655010, 49.65701158161629536 ) ) ;
#5131=AXIS2_PLACEMENT_3D ( 'NONE', #8025, #16594, #20044 ) ;
#5141=CARTESIAN_POINT ( 'NONE',  ( 0.000000000000000000, -126.9891397928655010, 0.000000000000000000 ) ) ;
#5145=DIRECTION ( 'NONE',  ( -0.000000000000000000, -0.000000000000000000, 1.000000000000000000 ) ) ;
#5146=CYLINDRICAL_SURFACE ( 'NONE', #15990, 10.00000000000000888 ) ;
#5164=EDGE_CURVE ( 'NONE', #12681, #6453, #21307, .T. ) ;
#5167=VECTOR ( 'NONE', #18512, 1000.000000000000000 ) ;
#5174=LINE ( 'NONE', #13652, #5553 ) ;
#5199=VECTOR ( 'NONE', #4218, 1000.000000000000000 ) ;
#5202=EDGE_CURVE ( 'NONE', #20722, #17644, #9409, .T. ) ;
#5207=CIRCLE ( 'NONE', #18926, 10.00000000000000888 ) ;
#5215=VERTEX_POINT ( 'NONE', #3113 ) ;
#5229=DIRECTION ( 'NONE',  ( 0.5010362705417046314, -0.000000000000000000, -0.8654262854811262118 ) ) ;
#5230=FACE_OUTER_BOUND ( 'NONE', #13458, .T. ) ;
#5232=CARTESIAN_POINT ( 'NONE',  ( 147.8787791192428074, -136.9891397928655010, 49.65701158161629536 ) ) ;
#5238=DIRECTION ( 'NONE',  ( -0.8302490056034136368, -0.5573926701119623628, 0.000000000000000000 ) ) ;
#5240=ORIENTED_EDGE ( 'NONE', *, *, #315, .F. ) ;
#5252=DIRECTION ( 'NONE',  ( 0.000000000000000000, -1.000000000000000000, 0.000000000000000000 ) ) ;
#5254=DIRECTION ( 'NONE',  ( 0.000000000000000000, -1.000000000000000000, 0.000000000000000000 ) ) ;
#5263=EDGE_CURVE ( 'NONE', #417, #2203, #13289, .T. ) ;
#5296=VERTEX_POINT ( 'NONE', #19530 ) ;
#5336=LINE ( 'NONE', #7004, #12375 ) ;
#5353=VECTOR ( 'NONE', #2562, 1000.000000000000000 ) ;
#5354=VECTOR ( 'NONE', #4513, 1000.000000000000000 ) ;
#5409=DIRECTION ( 'NONE',  ( 0.000000000000000000, -1.000000000000000000, 0.000000000000000000 ) ) ;
#5414=ORIENTED_EDGE ( 'NONE', *, *, #6178, .F. ) ;
#5418=ORIENTED_EDGE ( 'NONE', *, *, #19865, .F. ) ;
#5434=LINE ( 'NONE', #5123, #13226 ) ;
#5435=DIRECTION ( 'NONE',  ( 0.000000000000000000, 0.000000000000000000, 1.000000000000000000 ) ) ;
#5457=SHAPE_REPRESENTATION ( 'Cast Steel Heavy Body Block', ( #12657 ), #7388 ) ;
#5486=LINE ( 'NONE', #1866, #2344 ) ;
#5493=VECTOR ( 'NONE', #16535, 1000.000000000000000 ) ;
#5497=CIRCLE ( 'NONE', #16044, 7.500000000000000000 ) ;
#5500=CARTESIAN_POINT ( 'NONE',  ( 173.3794444120442506, -126.9891397928655010, 67.64809332337412684 ) ) ;
#5503=VECTOR ( 'NONE', #16954, 1000.000000000000000 ) ;
#5509=CARTESIAN_POINT ( 'NONE',  ( 91.17254549292282206, -61.68114226949890622, 30.00000000000000000 ) ) ;
#5533=CIRCLE ( 'NONE', #13986, 7.500000000000007105 ) ;
#5545=CARTESIAN_POINT ( 'NONE',  ( -88.69383338279318707, 132.1114735047150646, -35.00000000000000000 ) ) ;
#5553=VECTOR ( 'NONE', #18835, 1000.000000000000000 ) ;
#5592=DIRECTION ( 'NONE',  ( 0.000000000000000000, -1.000000000000000000, 0.000000000000000000 ) ) ;
#5598=VECTOR ( 'NONE', #16512, 1000.000000000000000 ) ;
#5601=VECTOR ( 'NONE', #9019, 1000.000000000000000 ) ;
#5605=DIRECTION ( 'NONE',  ( 0.000000000000000000, -1.000000000000000000, 0.000000000000000000 ) ) ;
#5611=ORIENTED_EDGE ( 'NONE', *, *, #15022, .F. ) ;
#5639=ORIENTED_EDGE ( 'NONE', *, *, #12879, .T. ) ;
#5650=CYLINDRICAL_SURFACE ( 'NONE', #17032, 10.00000000000000888 ) ;
#5667=VERTEX_POINT ( 'NONE', #15554 ) ;
#5688=FACE_OUTER_BOUND ( 'NONE', #12938, .T. ) ;
#5689=EDGE_LOOP ( 'NONE', ( #15384, #14421, #8334, #5639, #2466, #13181 ) ) ;
#5722=ORIENTED_EDGE ( 'NONE', *, *, #6927, .T. ) ;
#5723=DIRECTION ( 'NONE',  ( 2.779543948608941985E-16, -1.000000000000000000, 0.000000000000000000 ) ) ;
#5732=DIRECTION ( 'NONE',  ( 1.000000000000000000, 0.000000000000000000, 0.000000000000000000 ) ) ;
#5733=EDGE_CURVE ( 'NONE', #4745, #14655, #3280, .T. ) ;
#5747=ORIENTED_EDGE ( 'NONE', *, *, #10121, .F. ) ;
#5750=CARTESIAN_POINT ( 'NONE',  ( 173.3794444120442222, -37.13255853780189852, 19.99999999999999645 ) ) ;
#5758=UNCERTAINTY_MEASURE_WITH_UNIT (LENGTH_MEASURE( 1.000000000000000082E-05 ), #9575, 'distance_accuracy_value', 'NONE');
#5760=CARTESIAN_POINT ( 'NONE',  ( -120.0322075325610598, -126.9891397928655010, -34.99999999999999289 ) ) ;
#5774=ORIENTED_EDGE ( 'NONE', *, *, #12879, .F. ) ;
#5777=DIRECTION ( 'NONE',  ( -0.000000000000000000, -0.000000000000000000, 1.000000000000000000 ) ) ;
#5781=DIRECTION ( 'NONE',  ( -0.000000000000000000, -0.000000000000000000, 1.000000000000000000 ) ) ;
#5782=DIRECTION ( 'NONE',  ( 1.000000000000000000, 0.000000000000000000, 0.000000000000000000 ) ) ;
#5791=DIRECTION ( 'NONE',  ( 0.000000000000000000, 0.000000000000000000, 1.000000000000000000 ) ) ;
#5800=CARTESIAN_POINT ( 'NONE',  ( 18.67254549292281141, -61.68114226949890622, 20.00000000000000355 ) ) ;
#5808=CARTESIAN_POINT ( 'NONE',  ( -176.9699209214867608, 160.7104996726487514, -35.00000000000000000 ) ) ;
#5817=DIRECTION ( 'NONE',  ( -0.000000000000000000, 1.000000000000000000, -0.000000000000000000 ) ) ;
#5823=ADVANCED_FACE ( 'NONE', ( #12678 ), #4624, .F. ) ;
#5843=CYLINDRICAL_SURFACE ( 'NONE', #4636, 10.00000000000000888 ) ;
#5853=AXIS2_PLACEMENT_3D ( 'NONE', #19062, #10687, #7389 ) ;
#5887=CARTESIAN_POINT ( 'NONE',  ( -120.0322075325610598, -126.9891397928655010, -54.65701158161630246 ) ) ;
#5891=CARTESIAN_POINT ( 'NONE',  ( 11.17254549292281318, -61.68114226949890622, 30.00000000000000000 ) ) ;
#5901=DIRECTION ( 'NONE',  ( -0.000000000000000000, -0.000000000000000000, 1.000000000000000000 ) ) ;
#5911=ORIENTED_EDGE ( 'NONE', *, *, #8916, .T. ) ;
#5926=SURFACE_STYLE_USAGE ( .BOTH. , #2616 ) ;
#5963=ORIENTED_EDGE ( 'NONE', *, *, #10314, .T. ) ;
#5967=DIRECTION ( 'NONE',  ( 0.000000000000000000, -1.000000000000000000, 0.000000000000000000 ) ) ;
#5986=FACE_OUTER_BOUND ( 'NONE', #1665, .T. ) ;
#6015=VERTEX_POINT ( 'NONE', #4145 ) ;
#6028=CARTESIAN_POINT ( 'NONE',  ( 147.8787791192428074, -136.9891397928655010, 0.3429884183836981459 ) ) ;
#6045=DIRECTION ( 'NONE',  ( 0.000000000000000000, 0.000000000000000000, 1.000000000000000000 ) ) ;
#6095=ORIENTED_EDGE ( 'NONE', *, *, #26, .T. ) ;
#6103=DIRECTION ( 'NONE',  ( 1.000000000000000000, -0.000000000000000000, -0.000000000000000000 ) ) ;
#6106=DIRECTION ( 'NONE',  ( 1.000000000000000000, 0.000000000000000000, 0.000000000000000000 ) ) ;
#6122=ORIENTED_EDGE ( 'NONE', *, *, #17933, .F. ) ;
#6125=VECTOR ( 'NONE', #15117, 1000.000000000000000 ) ;
#6134=DIRECTION ( 'NONE',  ( -1.000000000000000000, -0.000000000000000000, -0.000000000000000000 ) ) ;
#6135=CARTESIAN_POINT ( 'NONE',  ( 101.4021762516569822, 137.5714195593754710, -35.00000000000000000 ) ) ;
#6139=DIRECTION ( 'NONE',  ( -0.000000000000000000, 0.000000000000000000, -1.000000000000000000 ) ) ;
#6147=VERTEX_POINT ( 'NONE', #2719 ) ;
#6175=ORIENTED_EDGE ( 'NONE', *, *, #10481, .F. ) ;
#6176=VERTEX_POINT ( 'NONE', #16592 ) ;
#6178=EDGE_CURVE ( 'NONE', #19406, #6147, #418, .T. ) ;
#6180=ORIENTED_EDGE ( 'NONE', *, *, #1690, .T. ) ;
#6188=CARTESIAN_POINT ( 'NONE',  ( 147.8787791192428074, -126.9891397928655010, 0.3429884183836981459 ) ) ;
#6191=EDGE_CURVE ( 'NONE', #21705, #13430, #7912, .T. ) ;
#6199=AXIS2_PLACEMENT_3D ( 'NONE', #19835, #4616, #11337 ) ;
#6200=ORIENTED_EDGE ( 'NONE', *, *, #929, .T. ) ;
#6227=VERTEX_POINT ( 'NONE', #16375 ) ;
#6228=FACE_BOUND ( 'NONE', #4406, .T. ) ;
#6238=CARTESIAN_POINT ( 'NONE',  ( 0.000000000000000000, -37.13255853780189852, 30.00000000000000000 ) ) ;
#6315=ORIENTED_EDGE ( 'NONE', *, *, #20512, .T. ) ;
#6352=CARTESIAN_POINT ( 'NONE',  ( -151.4692556286852891, -126.9891397928655010, 59.65701158161632378 ) ) ;
#6359=AXIS2_PLACEMENT_3D ( 'NONE', #21368, #1302, #9582 ) ;
#6360=CARTESIAN_POINT ( 'NONE',  ( -120.0322075325610598, -126.9891397928655010, -34.99999999999999289 ) ) ;
#6375=CARTESIAN_POINT ( 'NONE',  ( 173.3794444120442506, -37.13255853780189852, 30.00000000000000000 ) ) ;
#6382=LINE ( 'NONE', #13112, #4461 ) ;
#6387=LINE ( 'NONE', #1760, #2740 ) ;
#6402=EDGE_LOOP ( 'NONE', ( #847, #658 ) ) ;
#6453=VERTEX_POINT ( 'NONE', #16707 ) ;
#6460=ORIENTED_EDGE ( 'NONE', *, *, #9801, .F. ) ;
#6477=CIRCLE ( 'NONE', #1898, 27.58651506682278765 ) ;
#6493=EDGE_CURVE ( 'NONE', #9727, #9693, #2880, .T. ) ;
#6526=EDGE_CURVE ( 'NONE', #6147, #21749, #19338, .T. ) ;
#6531=DIRECTION ( 'NONE',  ( -0.000000000000000000, 0.000000000000000000, -1.000000000000000000 ) ) ;
#6544=EDGE_LOOP ( 'NONE', ( #10737, #15683 ) ) ;
#6555=DIRECTION ( 'NONE',  ( 0.5010362705417044094, 0.000000000000000000, -0.8654262854811263228 ) ) ;
#6558=EDGE_CURVE ( 'NONE', #11465, #11702, #15704, .T. ) ;
#6560=CARTESIAN_POINT ( 'NONE',  ( -47.86331837773882825, 0.000000000000000000, -35.00000000000000000 ) ) ;
#6572=EDGE_CURVE ( 'NONE', #6015, #14746, #19235, .T. ) ;
#6573=CARTESIAN_POINT ( 'NONE',  ( 156.1725454929228079, -61.68114226949890622, 19.99999999999998934 ) ) ;
#6578=ORIENTED_EDGE ( 'NONE', *, *, #13365, .F. ) ;
#6617=CARTESIAN_POINT ( 'NONE',  ( 173.3794444120442506, -126.9891397928655010, 30.00000000000000000 ) ) ;
#6626=VECTOR ( 'NONE', #13316, 1000.000000000000000 ) ;
#6629=VECTOR ( 'NONE', #18124, 1000.000000000000000 ) ;
#6640=ORIENTED_EDGE ( 'NONE', *, *, #15281, .F. ) ;
#6643=ORIENTED_EDGE ( 'NONE', *, *, #13573, .F. ) ;
#6650=AXIS2_PLACEMENT_3D ( 'NONE', #10707, #16681, #8215 ) ;
#6677=CARTESIAN_POINT ( 'NONE',  ( -120.0322075325610740, -136.9891397928655010, 49.65701158161630957 ) ) ;
#6680=DIRECTION ( 'NONE',  ( 0.000000000000000000, 0.000000000000000000, 1.000000000000000000 ) ) ;
#6684=CIRCLE ( 'NONE', #12641, 10.00000000000000888 ) ;
#6721=ORIENTED_EDGE ( 'NONE', *, *, #6806, .F. ) ;
#6754=CARTESIAN_POINT ( 'NONE',  ( -130.4480969619998234, -126.9891397928655010, 67.64809332337415526 ) ) ;
#6764=DIRECTION ( 'NONE',  ( -0.000000000000000000, -0.000000000000000000, -1.000000000000000000 ) ) ;
#6765=ORIENTED_EDGE ( 'NONE', *, *, #6572, .F. ) ;
#6778=EDGE_LOOP ( 'NONE', ( #3323, #4299, #3378, #21486 ) ) ;
#6785=AXIS2_PLACEMENT_3D ( 'NONE', #5500, #657, #3755 ) ;
#6806=EDGE_CURVE ( 'NONE', #9507, #119, #14807, .T. ) ;
#6809=EDGE_CURVE ( 'NONE', #2742, #11679, #14504, .T. ) ;
#6825=ORIENTED_EDGE ( 'NONE', *, *, #10439, .F. ) ;
#6829=CARTESIAN_POINT ( 'NONE',  ( -88.69383338279318707, 132.1114735047150646, -25.00000000000000000 ) ) ;
#6837=DIRECTION ( 'NONE',  ( 0.000000000000000000, 0.000000000000000000, -1.000000000000000000 ) ) ;
#6840=LINE ( 'NONE', #1542, #10497 ) ;
#6850=ORIENTED_EDGE ( 'NONE', *, *, #11475, .F. ) ;
#6862=PLANE ( 'NONE',  #9020 ) ;
#6867=ORIENTED_EDGE ( 'NONE', *, *, #6558, .F. ) ;
#6880=EDGE_LOOP ( 'NONE', ( #20103, #284, #11378, #18183 ) ) ;
#6902=ORIENTED_EDGE ( 'NONE', *, *, #17559, .F. ) ;
#6908=EDGE_LOOP ( 'NONE', ( #17800, #11088, #17201, #12718 ) ) ;
#6918=FACE_OUTER_BOUND ( 'NONE', #4524, .T. ) ;
#6927=EDGE_CURVE ( 'NONE', #15878, #15277, #17005, .T. ) ;
#6929=CARTESIAN_POINT ( 'NONE',  ( -176.9699209214867324, -136.9891397928655010, -72.64809332337415526 ) ) ;
#6965=LINE ( 'NONE', #6754, #17803 ) ;
#6978=VECTOR ( 'NONE', #9315, 1000.000000000000000 ) ;
#6981=ORIENTED_EDGE ( 'NONE', *, *, #593, .T. ) ;
#7004=CARTESIAN_POINT ( 'NONE',  ( 173.3794444120442506, -136.9891397928655010, 30.00000000000000000 ) ) ;
#7016=ORIENTED_EDGE ( 'NONE', *, *, #18390, .T. ) ;
#7039=EDGE_CURVE ( 'NONE', #6176, #2574, #8040, .T. ) ;
#7050=DIRECTION ( 'NONE',  ( 0.000000000000000000, 0.000000000000000000, 1.000000000000000000 ) ) ;
#7058=FACE_BOUND ( 'NONE', #16559, .T. ) ;
#7085=EDGE_LOOP ( 'NONE', ( #1463, #8666, #18935, #12489 ) ) ;
#7089=ORIENTED_EDGE ( 'NONE', *, *, #19577, .F. ) ;
#7094=ORIENTED_EDGE ( 'NONE', *, *, #5263, .T. ) ;
#7095=EDGE_CURVE ( 'NONE', #5296, #1608, #21772, .T. ) ;
#7109=PLANE ( 'NONE',  #7667 ) ;
#7116=VERTEX_POINT ( 'NONE', #4084 ) ;
#7129=CARTESIAN_POINT ( 'NONE',  ( 43.01140435219951996, 119.9070776186055838, -35.00000000000000000 ) ) ;
#7131=LINE ( 'NONE', #5887, #684 ) ;
#7171=CARTESIAN_POINT ( 'NONE',  ( 148.6725454929228079, -61.68114226949890622, 30.00000000000000000 ) ) ;
#7173=ORIENTED_EDGE ( 'NONE', *, *, #7768, .F. ) ;
#7192=EDGE_LOOP ( 'NONE', ( #247, #6095, #16178, #3883 ) ) ;
#7206=PLANE ( 'NONE',  #14231 ) ;
#7210=AXIS2_PLACEMENT_3D ( 'NONE', #13862, #2082, #11995 ) ;
#7216=DIRECTION ( 'NONE',  ( 0.000000000000000000, 0.000000000000000000, 1.000000000000000000 ) ) ;
#7232=VERTEX_POINT ( 'NONE', #18290 ) ;
#7252=ORIENTED_EDGE ( 'NONE', *, *, #9356, .F. ) ;
#7287=VECTOR ( 'NONE', #3110, 1000.000000000000000 ) ;
#7296=VECTOR ( 'NONE', #21107, 1000.000000000000000 ) ;
#7299=LINE ( 'NONE', #12344, #9017 ) ;
#7306=ADVANCED_FACE ( 'NONE', ( #3193 ), #8380, .T. ) ;
#7319=VECTOR ( 'NONE', #13142, 1000.000000000000000 ) ;
#7326=EDGE_CURVE ( 'NONE', #14746, #11386, #11446, .T. ) ;
#7335=AXIS2_PLACEMENT_3D ( 'NONE', #8477, #17042, #11760 ) ;
#7338=CARTESIAN_POINT ( 'NONE',  ( -151.4692556286852891, -126.9891397928655010, -44.65701158161626694 ) ) ;
#7339=DIRECTION ( 'NONE',  ( -0.8302490056034136368, -0.5573926701119623628, 9.854660648260997410E-17 ) ) ;
#7342=ORIENTED_EDGE ( 'NONE', *, *, #5733, .T. ) ;
#7343=PLANE ( 'NONE',  #590 ) ;
#7345=CARTESIAN_POINT ( 'NONE',  ( -120.0322075325610740, -126.9891397928655010, 30.00000000000000000 ) ) ;
#7388=( GEOMETRIC_REPRESENTATION_CONTEXT ( 3 ) GLOBAL_UNCERTAINTY_ASSIGNED_CONTEXT ( ( #2663 ) ) GLOBAL_UNIT_ASSIGNED_CONTEXT ( ( #12101, #3953, #14187 ) ) REPRESENTATION_CONTEXT ( 'NONE', 'WORKASPACE' ) );
#7389=DIRECTION ( 'NONE',  ( 1.000000000000000000, 0.000000000000000000, 0.000000000000000000 ) ) ;
#7450=FACE_OUTER_BOUND ( 'NONE', #16031, .T. ) ;
#7455=CARTESIAN_POINT ( 'NONE',  ( 111.4021762516569964, 137.5714195593754710, -35.00000000000000000 ) ) ;
#7469=VECTOR ( 'NONE', #6764, 1000.000000000000000 ) ;
#7474=ADVANCED_FACE ( 'NONE', ( #18620 ), #12100, .F. ) ;
#7477=DIRECTION ( 'NONE',  ( 0.5573926701119623628, -0.8302490056034136368, 0.000000000000000000 ) ) ;
#7478=ADVANCED_FACE ( 'NONE', ( #20708 ), #13969, .T. ) ;
#7485=VECTOR ( 'NONE', #2625, 1000.000000000000000 ) ;
#7486=CARTESIAN_POINT ( 'NONE',  ( 144.5586921005913439, 133.1239846058259388, -35.00000000000000000 ) ) ;
#7491=VECTOR ( 'NONE', #19667, 1000.000000000000000 ) ;
#7498=FACE_OUTER_BOUND ( 'NONE', #17738, .T. ) ;
#7502=PLANE ( 'NONE',  #6785 ) ;
#7526=ORIENTED_EDGE ( 'NONE', *, *, #15389, .F. ) ;
#7530=DIRECTION ( 'NONE',  ( 0.000000000000000000, 0.000000000000000000, 1.000000000000000000 ) ) ;
#7587=EDGE_CURVE ( 'NONE', #20193, #11386, #16959, .T. ) ;
#7590=ADVANCED_FACE ( 'NONE', ( #7058, #15631, #328 ), #437, .T. ) ;
#7612=VECTOR ( 'NONE', #3396, 1000.000000000000227 ) ;
#7617=DIRECTION ( 'NONE',  ( -0.000000000000000000, -0.000000000000000000, 1.000000000000000000 ) ) ;
#7631=DIRECTION ( 'NONE',  ( 0.000000000000000000, -1.000000000000000000, 0.000000000000000000 ) ) ;
#7648=MANIFOLD_SOLID_BREP ( 'Boss-Extrude14', #8831 ) ;
#7653=VECTOR ( 'NONE', #14968, 1000.000000000000000 ) ;
#7658=VERTEX_POINT ( 'NONE', #14193 ) ;
#7667=AXIS2_PLACEMENT_3D ( 'NONE', #17117, #160, #5435 ) ;
#7668=ORIENTED_EDGE ( 'NONE', *, *, #6572, .T. ) ;
#7679=CARTESIAN_POINT ( 'NONE',  ( 83.67254549292280785, -61.68114226949890622, -46.21320343559645494 ) ) ;
#7680=LINE ( 'NONE', #19027, #15673 ) ;
#7688=AXIS2_PLACEMENT_3D ( 'NONE', #9651, #16352, #6680 ) ;
#7697=ORIENTED_EDGE ( 'NONE', *, *, #3159, .F. ) ;
#7714=DIRECTION ( 'NONE',  ( 0.000000000000000000, 0.000000000000000000, 1.000000000000000000 ) ) ;
#7729=VECTOR ( 'NONE', #11410, 1000.000000000000000 ) ;
#7759=DIRECTION ( 'NONE',  ( 1.000000000000000000, 0.000000000000000000, -1.257660470541341077E-16 ) ) ;
#7768=EDGE_CURVE ( 'NONE', #3989, #6015, #16827, .T. ) ;
#7814=PLANE ( 'NONE',  #19777 ) ;
#7815=AXIS2_PLACEMENT_3D ( 'NONE', #8746, #12036, #20319 ) ;
#7820=VECTOR ( 'NONE', #16161, 1000.000000000000000 ) ;
#7873=ORIENTED_EDGE ( 'NONE', *, *, #11424, .F. ) ;
#7898=EDGE_LOOP ( 'NONE', ( #11171, #6643, #15658, #3321 ) ) ;
#7912=LINE ( 'NONE', #9786, #7820 ) ;
#7916=CARTESIAN_POINT ( 'NONE',  ( -176.9699209214867608, -126.9891397928655010, 67.64809332337415526 ) ) ;
#7922=LINE ( 'NONE', #2838, #6626 ) ;
#7923=DIRECTION ( 'NONE',  ( -1.000000000000000000, 0.000000000000000000, 0.000000000000000000 ) ) ;
#7974=ORIENTED_EDGE ( 'NONE', *, *, #17933, .T. ) ;
#7981=AXIS2_PLACEMENT_3D ( 'NONE', #15026, #151, #10193 ) ;
#7982=EDGE_CURVE ( 'NONE', #10538, #20193, #18381, .T. ) ;
#7998=DIRECTION ( 'NONE',  ( -1.140132994654635861E-16, -0.000000000000000000, -1.000000000000000000 ) ) ;
#8007=CARTESIAN_POINT ( 'NONE',  ( 33.01140435219951286, 119.9070776186055838, -35.00000000000000000 ) ) ;
#8019=ADVANCED_FACE ( 'NONE', ( #5688 ), #943, .F. ) ;
#8020=AXIS2_PLACEMENT_3D ( 'NONE', #49, #17011, #11727 ) ;
#8025=CARTESIAN_POINT ( 'NONE',  ( 111.4021762516569964, 137.5714195593754710, -35.00000000000000000 ) ) ;
#8038=EDGE_CURVE ( 'NONE', #7658, #19406, #6477, .T. ) ;
#8040=CIRCLE ( 'NONE', #6650, 10.00000000000000888 ) ;
#8041=EDGE_LOOP ( 'NONE', ( #4541, #4091, #16197, #8955, #21027, #16222, #15590, #21733, #20879, #1225, #8451, #2175, #17182, #20537, #15801, #16723, #12711, #20352 ) ) ;
#8072=AXIS2_PLACEMENT_3D ( 'NONE', #5800, #10565, #2280 ) ;
#8077=DIRECTION ( 'NONE',  ( -0.000000000000000000, -0.000000000000000000, 1.000000000000000000 ) ) ;
#8078=DIRECTION ( 'NONE',  ( -0.000000000000000000, -0.000000000000000000, -1.000000000000000000 ) ) ;
#8079=DIRECTION ( 'NONE',  ( 1.000000000000000000, 0.000000000000000000, 0.000000000000000000 ) ) ;
#8089=DIRECTION ( 'NONE',  ( -1.000000000000000000, 0.000000000000000000, 0.000000000000000000 ) ) ;
#8099=DIRECTION ( 'NONE',  ( 0.8302490056034133037, 0.5573926701119628069, -0.000000000000000000 ) ) ;
#8112=ORIENTED_EDGE ( 'NONE', *, *, #11528, .F. ) ;
#8140=EDGE_CURVE ( 'NONE', #18529, #5215, #2814, .T. ) ;
#8144=ORIENTED_EDGE ( 'NONE', *, *, #5733, .F. ) ;
#8160=CARTESIAN_POINT ( 'NONE',  ( 144.5586921005913439, -37.13255853780189852, -19.99999999999999645 ) ) ;
#8180=EDGE_LOOP ( 'NONE', ( #3569, #6981, #14017, #16784, #14990, #8511, #17439, #14801 ) ) ;
#8200=ORIENTED_EDGE ( 'NONE', *, *, #5202, .T. ) ;
#8215=DIRECTION ( 'NONE',  ( 0.000000000000000000, 0.000000000000000000, 1.000000000000000000 ) ) ;
#8216=LINE ( 'NONE', #21665, #10983 ) ;
#8227=FACE_OUTER_BOUND ( 'NONE', #5689, .T. ) ;
#8236=DIRECTION ( 'NONE',  ( -0.000000000000000000, -0.000000000000000000, 1.000000000000000000 ) ) ;
#8256=ORIENTED_EDGE ( 'NONE', *, *, #593, .F. ) ;
#8265=EDGE_CURVE ( 'NONE', #1696, #11702, #633, .T. ) ;
#8286=VERTEX_POINT ( 'NONE', #8007 ) ;
#8292=EDGE_CURVE ( 'NONE', #7116, #5296, #20131, .T. ) ;
#8294=LINE ( 'NONE', #20096, #15341 ) ;
#8295=AXIS2_PLACEMENT_3D ( 'NONE', #16819, #13520, #20574 ) ;
#8327=CARTESIAN_POINT ( 'NONE',  ( -39.63192160874135084, -136.9891397928655010, 20.00000000000002132 ) ) ;
#8328=VECTOR ( 'NONE', #15622, 1000.000000000000000 ) ;
#8334=ORIENTED_EDGE ( 'NONE', *, *, #20907, .F. ) ;
#8350=DIRECTION ( 'NONE',  ( 0.000000000000000000, 0.000000000000000000, -1.000000000000000000 ) ) ;
#8380=PLANE ( 'NONE',  #11227 ) ;
#8381=DIRECTION ( 'NONE',  ( 0.000000000000000000, -1.000000000000000000, 0.000000000000000000 ) ) ;
#8409=LINE ( 'NONE', #4756, #7287 ) ;
#8423=EDGE_CURVE ( 'NONE', #6176, #15753, #4685, .T. ) ;
#8431=DIRECTION ( 'NONE',  ( 0.000000000000000000, 0.000000000000000000, 1.000000000000000000 ) ) ;
#8435=DIRECTION ( 'NONE',  ( 0.000000000000000000, -1.000000000000000000, 0.000000000000000000 ) ) ;
#8450=CARTESIAN_POINT ( 'NONE',  ( -130.4480969619998234, -136.9891397928655010, 67.64809332337415526 ) ) ;
#8451=ORIENTED_EDGE ( 'NONE', *, *, #8292, .T. ) ;
#8458=VERTEX_POINT ( 'NONE', #10095 ) ;
#8477=CARTESIAN_POINT ( 'NONE',  ( 126.8576204525573274, -126.9891397928655010, 67.64809332337412684 ) ) ;
#8511=ORIENTED_EDGE ( 'NONE', *, *, #14257, .T. ) ;
#8531=VERTEX_POINT ( 'NONE', #18896 ) ;
#8534=AXIS2_PLACEMENT_3D ( 'NONE', #13901, #20640, #11931 ) ;
#8544=VECTOR ( 'NONE', #19491, 1000.000000000000000 ) ;
#8611=VERTEX_POINT ( 'NONE', #8450 ) ;
#8645=AXIS2_PLACEMENT_3D ( 'NONE', #14055, #4343, #15812 ) ;
#8649=DIRECTION ( 'NONE',  ( 0.000000000000000000, 0.000000000000000000, 1.000000000000000000 ) ) ;
#8654=PLANE ( 'NONE',  #8020 ) ;
#8666=ORIENTED_EDGE ( 'NONE', *, *, #11528, .T. ) ;
#8684=PLANE ( 'NONE',  #7335 ) ;
#8746=CARTESIAN_POINT ( 'NONE',  ( 0.000000000000000000, -126.9891397928655010, 0.000000000000000000 ) ) ;
#8764=CARTESIAN_POINT ( 'NONE',  ( -176.9699209214867608, 160.7104996726487514, -35.00000000000000000 ) ) ;
#8805=LINE ( 'NONE', #2177, #5601 ) ;
#8815=CARTESIAN_POINT ( 'NONE',  ( 0.000000000000000000, -136.9891397928655010, 30.00000000000000000 ) ) ;
#8831=CLOSED_SHELL ( 'NONE', ( #8019, #19017, #9106, #19775, #9479, #15959, #19519, #11762, #10378, #677, #12731, #19566, #4874, #5823, #2774, #17783, #20611, #566, #14868, #19178, #16046, #21081, #11091, #21271, #2377, #4283, #18322, #7590, #3833, #7474, #9079, #20024, #4925, #2328, #16885, #4911, #17278, #7306, #17390, #18021, #2958, #18063, #14212, #21229, #1538, #7478, #3903, #14717, #516, #42 ) ) ;
#8843=EDGE_CURVE ( 'NONE', #16314, #1116, #8409, .T. ) ;
#8845=CARTESIAN_POINT ( 'NONE',  ( 116.4417310231185780, -136.9891397928655010, 0.3429884183836981459 ) ) ;
#8855=FACE_OUTER_BOUND ( 'NONE', #10457, .T. ) ;
#8872=VECTOR ( 'NONE', #11605, 1000.000000000000000 ) ;
#8893=CARTESIAN_POINT ( 'NONE',  ( 116.4417310231185780, -126.9891397928655010, 49.65701158161629536 ) ) ;
#8916=EDGE_CURVE ( 'NONE', #14655, #13351, #3291, .T. ) ;
#8919=CARTESIAN_POINT ( 'NONE',  ( 111.4021762516569964, 137.5714195593754710, -35.00000000000000000 ) ) ;
#8920=FACE_OUTER_BOUND ( 'NONE', #8041, .T. ) ;
#8934=PLANE ( 'NONE',  #19093 ) ;
#8935=ORIENTED_EDGE ( 'NONE', *, *, #11384, .T. ) ;
#8955=ORIENTED_EDGE ( 'NONE', *, *, #13552, .T. ) ;
#8957=PLANE ( 'NONE',  #8534 ) ;
#8969=STYLED_ITEM ( 'NONE', ( #14519 ), #7648 ) ;
#8994=CARTESIAN_POINT ( 'NONE',  ( -176.9699209214867608, -126.9891397928655010, 67.64809332337415526 ) ) ;
#9017=VECTOR ( 'NONE', #20520, 1000.000000000000000 ) ;
#9019=DIRECTION ( 'NONE',  ( 0.000000000000000000, -1.000000000000000000, 0.000000000000000000 ) ) ;
#9020=AXIS2_PLACEMENT_3D ( 'NONE', #13568, #6531, #1569 ) ;
#9028=FACE_BOUND ( 'NONE', #147, .T. ) ;
#9055=DIRECTION ( 'NONE',  ( 0.000000000000000000, -1.000000000000000000, 0.000000000000000000 ) ) ;
#9063=VECTOR ( 'NONE', #21548, 1000.000000000000000 ) ;
#9065=FACE_OUTER_BOUND ( 'NONE', #19114, .T. ) ;
#9067=EDGE_CURVE ( 'NONE', #11702, #1696, #5497, .T. ) ;
#9074=CIRCLE ( 'NONE', #15751, 10.00000000000000888 ) ;
#9079=ADVANCED_FACE ( 'NONE', ( #11369 ), #6862, .T. ) ;
#9083=DIRECTION ( 'NONE',  ( 1.000000000000000000, 0.000000000000000000, 0.000000000000000000 ) ) ;
#9106=ADVANCED_FACE ( 'NONE', ( #3332 ), #18433, .F. ) ;
#9131=CIRCLE ( 'NONE', #4549, 27.58651506682278765 ) ;
#9139=SHAPE_REPRESENTATION_RELATIONSHIP ( 'NONE' , 'NONE' ,  #5457, #2967 ) ;
#9168=CARTESIAN_POINT ( 'NONE',  ( 111.4021762516569964, 137.5714195593754710, -35.00000000000000000 ) ) ;
#9201=VERTEX_POINT ( 'NONE', #8845 ) ;
#9212=CARTESIAN_POINT ( 'NONE',  ( -39.63192160874135084, -354.7018910364275257, 20.00000000000002132 ) ) ;
#9239=CARTESIAN_POINT ( 'NONE',  ( 156.1725454929228079, -61.68114226949890622, -46.21320343559645494 ) ) ;
#9257=CARTESIAN_POINT ( 'NONE',  ( 132.3486983259487886, 110.2203079035326851, -19.99999999999999645 ) ) ;
#9260=ORIENTED_EDGE ( 'NONE', *, *, #12468, .T. ) ;
#9262=ORIENTED_EDGE ( 'NONE', *, *, #19692, .T. ) ;
#9278=EDGE_LOOP ( 'NONE', ( #21569, #1804 ) ) ;
#9288=ORIENTED_EDGE ( 'NONE', *, *, #20512, .F. ) ;
#9297=CARTESIAN_POINT ( 'NONE',  ( 148.6725454929228079, -61.68114226949890622, 30.00000000000000000 ) ) ;
#9308=DIRECTION ( 'NONE',  ( 0.000000000000000000, 0.000000000000000000, -1.000000000000000000 ) ) ;
#9309=AXIS2_PLACEMENT_3D ( 'NONE', #13782, #3983, #13890 ) ;
#9315=DIRECTION ( 'NONE',  ( -0.000000000000000000, 1.000000000000000000, -0.000000000000000000 ) ) ;
#9321=VECTOR ( 'NONE', #15920, 1000.000000000000000 ) ;
#9341=CARTESIAN_POINT ( 'NONE',  ( 173.3794444120442222, -136.9891397928655010, 19.99999999999999645 ) ) ;
#9350=DIRECTION ( 'NONE',  ( 1.000000000000000000, 0.000000000000000000, -0.000000000000000000 ) ) ;
#9356=EDGE_CURVE ( 'NONE', #8531, #9507, #2637, .T. ) ;
#9365=ORIENTED_EDGE ( 'NONE', *, *, #19858, .T. ) ;
#9389=DIRECTION ( 'NONE',  ( 0.000000000000000000, 0.000000000000000000, 1.000000000000000000 ) ) ;
#9394=ORIENTED_EDGE ( 'NONE', *, *, #12584, .T. ) ;
#9397=ORIENTED_EDGE ( 'NONE', *, *, #1934, .F. ) ;
#9405=DIRECTION ( 'NONE',  ( 0.000000000000000000, 0.000000000000000000, -1.000000000000000000 ) ) ;
#9409=LINE ( 'NONE', #14564, #11168 ) ;
#9416=EDGE_LOOP ( 'NONE', ( #6460, #14119, #19521, #5774 ) ) ;
#9446=AXIS2_PLACEMENT_3D ( 'NONE', #9168, #15867, #20953 ) ;
#9447=DIRECTION ( 'NONE',  ( 1.000000000000000000, 0.000000000000000000, 0.000000000000000000 ) ) ;
#9479=ADVANCED_FACE ( 'NONE', ( #17731 ), #19188, .F. ) ;
#9488=CARTESIAN_POINT ( 'NONE',  ( 11.17254549292281318, -61.68114226949890622, -46.21320343559645494 ) ) ;
#9500=ORIENTED_EDGE ( 'NONE', *, *, #10121, .T. ) ;
#9507=VERTEX_POINT ( 'NONE', #2536 ) ;
#9526=EDGE_CURVE ( 'NONE', #20108, #4552, #9816, .T. ) ;
#9570=LINE ( 'NONE', #7916, #20571 ) ;
#9575=( LENGTH_UNIT ( ) NAMED_UNIT ( * ) SI_UNIT ( .MILLI., .METRE. ) );
#9580=CARTESIAN_POINT ( 'NONE',  ( 173.3794444120442506, -126.9891397928655010, 67.64809332337412684 ) ) ;
#9582=DIRECTION ( 'NONE',  ( 0.000000000000000000, 0.000000000000000000, -1.000000000000000000 ) ) ;
#9590=AXIS2_PLACEMENT_3D ( 'NONE', #16063, #7714, #14415 ) ;
#9609=EDGE_CURVE ( 'NONE', #4967, #119, #4843, .T. ) ;
#9639=EDGE_CURVE ( 'NONE', #6227, #6453, #6387, .T. ) ;
#9651=CARTESIAN_POINT ( 'NONE',  ( 147.8787791192428074, -136.9891397928655010, 49.65701158161629536 ) ) ;
#9693=VERTEX_POINT ( 'NONE', #4960 ) ;
#9694=DIRECTION ( 'NONE',  ( 0.000000000000000000, 0.000000000000000000, 1.000000000000000000 ) ) ;
#9722=VERTEX_POINT ( 'NONE', #3081 ) ;
#9727=VERTEX_POINT ( 'NONE', #16514 ) ;
#9734=CARTESIAN_POINT ( 'NONE',  ( 148.6725454929228079, -61.68114226949890622, -46.21320343559645494 ) ) ;
#9756=EDGE_CURVE ( 'NONE', #18667, #20725, #5486, .T. ) ;
#9758=CARTESIAN_POINT ( 'NONE',  ( -39.63192160874127978, -354.7018910364275257, -35.00000000000000000 ) ) ;
#9762=DIRECTION ( 'NONE',  ( 0.000000000000000000, -1.000000000000000000, 0.000000000000000000 ) ) ;
#9776=VECTOR ( 'NONE', #14376, 1000.000000000000000 ) ;
#9782=PLANE ( 'NONE',  #1032 ) ;
#9786=CARTESIAN_POINT ( 'NONE',  ( 0.000000000000000000, -37.13255853780189852, -35.00000000000000000 ) ) ;
#9788=CIRCLE ( 'NONE', #17853, 7.500000000000007105 ) ;
#9801=EDGE_CURVE ( 'NONE', #6227, #4859, #12213, .T. ) ;
#9815=CARTESIAN_POINT ( 'NONE',  ( 116.4417310231185780, -126.9891397928655010, 30.00000000000000000 ) ) ;
#9816=LINE ( 'NONE', #20178, #5167 ) ;
#9829=ORIENTED_EDGE ( 'NONE', *, *, #12154, .F. ) ;
#9831=EDGE_CURVE ( 'NONE', #6147, #17644, #5174, .T. ) ;
#9834=CARTESIAN_POINT ( 'NONE',  ( -130.4480969619997950, -136.9891397928655010, -72.64809332337412684 ) ) ;
#9868=CARTESIAN_POINT ( 'NONE',  ( 148.6725454929228079, -61.68114226949890622, 19.99999999999998934 ) ) ;
#9889=FACE_BOUND ( 'NONE', #6544, .T. ) ;
#9932=EDGE_CURVE ( 'NONE', #20322, #16938, #11483, .T. ) ;
#9940=ORIENTED_EDGE ( 'NONE', *, *, #11768, .T. ) ;
#10010=DIRECTION ( 'NONE',  ( -0.5573926701119628069, 0.8302490056034133037, 0.000000000000000000 ) ) ;
#10018=CIRCLE ( 'NONE', #9309, 10.00000000000000888 ) ;
#10021=ORIENTED_EDGE ( 'NONE', *, *, #21370, .T. ) ;
#10036=DIRECTION ( 'NONE',  ( 1.000000000000000000, 0.000000000000000000, 0.000000000000000000 ) ) ;
#10043=VERTEX_POINT ( 'NONE', #21255 ) ;
#10052=ORIENTED_EDGE ( 'NONE', *, *, #10623, .T. ) ;
#10060=CARTESIAN_POINT ( 'NONE',  ( 116.4417310231185780, -136.9891397928655010, 19.99999999999999645 ) ) ;
#10061=CARTESIAN_POINT ( 'NONE',  ( -151.4692556286852891, -126.9891397928655010, -54.65701158161630246 ) ) ;
#10070=VERTEX_POINT ( 'NONE', #6135 ) ;
#10095=CARTESIAN_POINT ( 'NONE',  ( 173.3794444120442506, -136.9891397928655010, 67.64809332337412684 ) ) ;
#10121=EDGE_CURVE ( 'NONE', #706, #8458, #20570, .T. ) ;
#10152=ORIENTED_EDGE ( 'NONE', *, *, #11384, .F. ) ;
#10158=EDGE_CURVE ( 'NONE', #8286, #18069, #17817, .T. ) ;
#10188=ORIENTED_EDGE ( 'NONE', *, *, #19858, .F. ) ;
#10193=DIRECTION ( 'NONE',  ( 0.000000000000000000, 0.000000000000000000, -1.000000000000000000 ) ) ;
#10211=CARTESIAN_POINT ( 'NONE',  ( 116.4417310231185780, -126.9891397928655010, 19.99999999999999645 ) ) ;
#10220=DIRECTION ( 'NONE',  ( 0.000000000000000000, 0.000000000000000000, 1.000000000000000000 ) ) ;
#10238=ORIENTED_EDGE ( 'NONE', *, *, #12053, .F. ) ;
#10243=AXIS2_PLACEMENT_3D ( 'NONE', #12661, #14200, #15637 ) ;
#10262=DIRECTION ( 'NONE',  ( 1.000000000000000000, 0.000000000000000000, 0.000000000000000000 ) ) ;
#10277=DIRECTION ( 'NONE',  ( 0.000000000000000000, 0.000000000000000000, -1.000000000000000000 ) ) ;
#10304=PLANE ( 'NONE',  #2188 ) ;
#10306=DIRECTION ( 'NONE',  ( 0.000000000000000000, -1.000000000000000000, 0.000000000000000000 ) ) ;
#10314=EDGE_CURVE ( 'NONE', #19403, #20725, #21360, .T. ) ;
#10333=CARTESIAN_POINT ( 'NONE',  ( 147.8787791192428074, -126.9891397928655010, 0.3429884183836981459 ) ) ;
#10358=VECTOR ( 'NONE', #5901, 1000.000000000000000 ) ;
#10375=CARTESIAN_POINT ( 'NONE',  ( -176.9699209214867892, -4.918956727831215833E-14, 30.00000000000000000 ) ) ;
#10378=ADVANCED_FACE ( 'NONE', ( #7450 ), #19022, .F. ) ;
#10397=VERTEX_POINT ( 'NONE', #2258 ) ;
#10405=DIRECTION ( 'NONE',  ( -0.5010362705417046314, 0.000000000000000000, 0.8654262854811262118 ) ) ;
#10407=VECTOR ( 'NONE', #1631, 1000.000000000000000 ) ;
#10423=ORIENTED_EDGE ( 'NONE', *, *, #8292, .F. ) ;
#10424=LINE ( 'NONE', #16913, #12935 ) ;
#10439=EDGE_CURVE ( 'NONE', #735, #5296, #609, .T. ) ;
#10451=VECTOR ( 'NONE', #5252, 1000.000000000000000 ) ;
#10457=EDGE_LOOP ( 'NONE', ( #21244, #1899, #10052, #10021 ) ) ;
#10464=VECTOR ( 'NONE', #8099, 1000.000000000000114 ) ;
#10481=EDGE_CURVE ( 'NONE', #6227, #13430, #4781, .T. ) ;
#10497=VECTOR ( 'NONE', #20180, 1000.000000000000000 ) ;
#10514=CARTESIAN_POINT ( 'NONE',  ( 173.3794444120442506, -126.9891397928655010, 19.99999999999999645 ) ) ;
#10516=LINE ( 'NONE', #17646, #19575 ) ;
#10525=CARTESIAN_POINT ( 'NONE',  ( 116.4417310231185780, -126.9891397928655010, 19.99999999999999645 ) ) ;
#10529=DIRECTION ( 'NONE',  ( 0.000000000000000000, 0.000000000000000000, 1.000000000000000000 ) ) ;
#10531=ORIENTED_EDGE ( 'NONE', *, *, #1934, .T. ) ;
#10538=VERTEX_POINT ( 'NONE', #3022 ) ;
#10546=CYLINDRICAL_SURFACE ( 'NONE', #8295, 10.00000000000000888 ) ;
#10557=EDGE_CURVE ( 'NONE', #18667, #7658, #11176, .T. ) ;
#10565=DIRECTION ( 'NONE',  ( -1.140132994654635861E-16, -0.000000000000000000, -1.000000000000000000 ) ) ;
#10573=FACE_BOUND ( 'NONE', #5055, .T. ) ;
#10618=DIRECTION ( 'NONE',  ( 1.000000000000000000, 0.000000000000000000, 0.000000000000000000 ) ) ;
#10623=EDGE_CURVE ( 'NONE', #16314, #17801, #18111, .T. ) ;
#10631=CARTESIAN_POINT ( 'NONE',  ( 116.4417310231185780, -126.9891397928655010, 0.3429884183836981459 ) ) ;
#10638=ORIENTED_EDGE ( 'NONE', *, *, #20781, .T. ) ;
#10651=VECTOR ( 'NONE', #5229, 1000.000000000000000 ) ;
#10664=ORIENTED_EDGE ( 'NONE', *, *, #3564, .F. ) ;
#10679=FACE_BOUND ( 'NONE', #13098, .T. ) ;
#10687=DIRECTION ( 'NONE',  ( 0.000000000000000000, 0.000000000000000000, 1.000000000000000000 ) ) ;
#10707=CARTESIAN_POINT ( 'NONE',  ( 147.8787791192428074, -126.9891397928655010, 49.65701158161629536 ) ) ;
#10714=EDGE_LOOP ( 'NONE', ( #4667, #6825, #11939, #16128 ) ) ;
#10727=LINE ( 'NONE', #5750, #1997 ) ;
#10737=ORIENTED_EDGE ( 'NONE', *, *, #2276, .T. ) ;
#10748=ORIENTED_EDGE ( 'NONE', *, *, #17540, .T. ) ;
#10758=DIRECTION ( 'NONE',  ( 0.000000000000000000, 0.000000000000000000, 1.000000000000000000 ) ) ;
#10778=VECTOR ( 'NONE', #11621, 1000.000000000000000 ) ;
#10787=CYLINDRICAL_SURFACE ( 'NONE', #21652, 7.500000000000007105 ) ;
#10812=DIRECTION ( 'NONE',  ( 0.8302490056034133037, 0.5573926701119628069, -9.854660648260994945E-17 ) ) ;
#10825=VECTOR ( 'NONE', #10812, 1000.000000000000114 ) ;
#10832=ORIENTED_EDGE ( 'NONE', *, *, #15168, .T. ) ;
#10861=VERTEX_POINT ( 'NONE', #5509 ) ;
#10867=DIRECTION ( 'NONE',  ( -0.000000000000000000, -0.000000000000000000, 1.000000000000000000 ) ) ;
#10869=DIRECTION ( 'NONE',  ( 7.372372188207634192E-16, 0.000000000000000000, -1.000000000000000000 ) ) ;
#10880=DIRECTION ( 'NONE',  ( 0.000000000000000000, 0.000000000000000000, -1.000000000000000000 ) ) ;
#10888=ORIENTED_EDGE ( 'NONE', *, *, #8038, .F. ) ;
#10906=DIRECTION ( 'NONE',  ( -0.5010362705417045204, -0.000000000000000000, 0.8654262854811263228 ) ) ;
#10911=CARTESIAN_POINT ( 'NONE',  ( 33.01140435219951286, 119.9070776186055838, -35.00000000000000000 ) ) ;
#10918=CYLINDRICAL_SURFACE ( 'NONE', #14677, 7.500000000000000000 ) ;
#10937=ORIENTED_EDGE ( 'NONE', *, *, #18933, .F. ) ;
#10945=DIRECTION ( 'NONE',  ( 0.000000000000000000, -1.000000000000000000, 0.000000000000000000 ) ) ;
#10955=ORIENTED_EDGE ( 'NONE', *, *, #1543, .F. ) ;
#10957=CARTESIAN_POINT ( 'NONE',  ( 147.8787791192428074, -126.9891397928655010, 0.3429884183836981459 ) ) ;
#10983=VECTOR ( 'NONE', #8649, 1000.000000000000000 ) ;
#11029=EDGE_LOOP ( 'NONE', ( #1093, #14471, #17991, #11197 ) ) ;
#11069=CIRCLE ( 'NONE', #1581, 7.500000000000007105 ) ;
#11088=ORIENTED_EDGE ( 'NONE', *, *, #18399, .T. ) ;
#11091=ADVANCED_FACE ( 'NONE', ( #11228 ), #10918, .F. ) ;
#11100=CARTESIAN_POINT ( 'NONE',  ( -176.9699209214867324, -126.9891397928655010, -72.64809332337415526 ) ) ;
#11115=ORIENTED_EDGE ( 'NONE', *, *, #9932, .T. ) ;
#11167=EDGE_CURVE ( 'NONE', #20725, #417, #4082, .T. ) ;
#11168=VECTOR ( 'NONE', #16435, 1000.000000000000000 ) ;
#11171=ORIENTED_EDGE ( 'NONE', *, *, #17447, .F. ) ;
#11173=AXIS2_PLACEMENT_3D ( 'NONE', #13429, #96, #1635 ) ;
#11176=LINE ( 'NONE', #16134, #10464 ) ;
#11197=ORIENTED_EDGE ( 'NONE', *, *, #4559, .F. ) ;
#11227=AXIS2_PLACEMENT_3D ( 'NONE', #19836, #3079, #13439 ) ;
#11228=FACE_OUTER_BOUND ( 'NONE', #15979, .T. ) ;
#11248=ORIENTED_EDGE ( 'NONE', *, *, #20679, .T. ) ;
#11250=EDGE_CURVE ( 'NONE', #14746, #7116, #1646, .T. ) ;
#11269=CARTESIAN_POINT ( 'NONE',  ( -39.63192160874135084, -37.13255853780189852, 20.00000000000002132 ) ) ;
#11274=VERTEX_POINT ( 'NONE', #18170 ) ;
#11302=LINE ( 'NONE', #9341, #7729 ) ;
#11323=ORIENTED_EDGE ( 'NONE', *, *, #21370, .F. ) ;
#11329=CIRCLE ( 'NONE', #20853, 10.00000000000000888 ) ;
#11337=DIRECTION ( 'NONE',  ( 1.000000000000000000, 0.000000000000000000, 0.000000000000000000 ) ) ;
#11350=CARTESIAN_POINT ( 'NONE',  ( -176.9699209214867892, -37.13255853780189852, -19.99999999999995737 ) ) ;
#11356=EDGE_CURVE ( 'NONE', #18451, #1608, #18402, .T. ) ;
#11369=FACE_OUTER_BOUND ( 'NONE', #6880, .T. ) ;
#11378=ORIENTED_EDGE ( 'NONE', *, *, #18933, .T. ) ;
#11384=EDGE_CURVE ( 'NONE', #21749, #20722, #6382, .T. ) ;
#11386=VERTEX_POINT ( 'NONE', #6617 ) ;
#11401=CARTESIAN_POINT ( 'NONE',  ( 147.8787791192428074, -126.9891397928655010, 39.65701158161628825 ) ) ;
#11410=DIRECTION ( 'NONE',  ( 1.000000000000000000, 0.000000000000000000, -1.140132994654635861E-16 ) ) ;
#11420=LINE ( 'NONE', #6360, #14938 ) ;
#11424=EDGE_CURVE ( 'NONE', #4573, #4975, #14503, .T. ) ;
#11428=CARTESIAN_POINT ( 'NONE',  ( -47.86331837773882825, 0.000000000000000000, -25.00000000000000000 ) ) ;
#11433=VECTOR ( 'NONE', #21009, 1000.000000000000000 ) ;
#11444=DIRECTION ( 'NONE',  ( 0.000000000000000000, 0.000000000000000000, 1.000000000000000000 ) ) ;
#11446=LINE ( 'NONE', #9815, #5598 ) ;
#11450=CARTESIAN_POINT ( 'NONE',  ( -47.86331837773882825, -19.06233958201669765, -35.00000000000000000 ) ) ;
#11462=ORIENTED_EDGE ( 'NONE', *, *, #12200, .F. ) ;
#11465=VERTEX_POINT ( 'NONE', #2748 ) ;
#11475=EDGE_CURVE ( 'NONE', #9722, #1696, #879, .T. ) ;
#11483=CIRCLE ( 'NONE', #3758, 10.00000000000000888 ) ;
#11488=CARTESIAN_POINT ( 'NONE',  ( 126.8576204525573274, -126.9891397928655010, -17.64809332337413750 ) ) ;
#11489=CIRCLE ( 'NONE', #3043, 10.00000000000000888 ) ;
#11503=CARTESIAN_POINT ( 'NONE',  ( -151.4692556286852891, -126.9891397928655010, -54.65701158161630246 ) ) ;
#11517=CARTESIAN_POINT ( 'NONE',  ( 173.3794444120442222, -354.7018910364275257, 19.99999999999999645 ) ) ;
#11528=EDGE_CURVE ( 'NONE', #10070, #9693, #15398, .T. ) ;
#11553=CARTESIAN_POINT ( 'NONE',  ( 147.8787791192428074, -126.9891397928655010, 49.65701158161629536 ) ) ;
#11592=DIRECTION ( 'NONE',  ( 0.000000000000000000, 0.000000000000000000, 1.000000000000000000 ) ) ;
#11605=DIRECTION ( 'NONE',  ( 0.000000000000000000, 0.000000000000000000, 1.000000000000000000 ) ) ;
#11621=DIRECTION ( 'NONE',  ( 0.000000000000000000, 1.000000000000000000, -0.000000000000000000 ) ) ;
#11654=ORIENTED_EDGE ( 'NONE', *, *, #8140, .F. ) ;
#11664=CARTESIAN_POINT ( 'NONE',  ( 116.4417310231185780, -126.9891397928655010, 30.00000000000000000 ) ) ;
#11667=VECTOR ( 'NONE', #5238, 1000.000000000000114 ) ;
#11679=VERTEX_POINT ( 'NONE', #18916 ) ;
#11686=EDGE_LOOP ( 'NONE', ( #13129, #113, #18897, #9365 ) ) ;
#11687=VECTOR ( 'NONE', #15033, 1000.000000000000000 ) ;
#11701=LINE ( 'NONE', #15121, #7469 ) ;
#11702=VERTEX_POINT ( 'NONE', #1840 ) ;
#11718=CARTESIAN_POINT ( 'NONE',  ( -39.63192160874127978, -37.13255853780189852, -35.00000000000000000 ) ) ;
#11727=DIRECTION ( 'NONE',  ( -0.000000000000000000, 0.000000000000000000, -1.000000000000000000 ) ) ;
#11734=CARTESIAN_POINT ( 'NONE',  ( 0.000000000000000000, -136.9891397928655010, 30.00000000000000000 ) ) ;
#11760=DIRECTION ( 'NONE',  ( 0.5010362705417047424, 0.000000000000000000, 0.8654262854811261008 ) ) ;
#11762=ADVANCED_FACE ( 'NONE', ( #21115 ), #724, .F. ) ;
#11766=AXIS2_PLACEMENT_3D ( 'NONE', #6188, #10945, #9405 ) ;
#11768=EDGE_CURVE ( 'NONE', #21314, #5667, #20786, .T. ) ;
#11792=LINE ( 'NONE', #114, #20140 ) ;
#11807=FACE_OUTER_BOUND ( 'NONE', #16859, .T. ) ;
#11811=CARTESIAN_POINT ( 'NONE',  ( 141.1725454929228079, -61.68114226949890622, 19.99999999999998934 ) ) ;
#11816=ORIENTED_EDGE ( 'NONE', *, *, #3276, .F. ) ;
#11834=EDGE_CURVE ( 'NONE', #15585, #11274, #14262, .T. ) ;
#11873=CARTESIAN_POINT ( 'NONE',  ( 126.8576204525573274, -126.9891397928655010, 67.64809332337412684 ) ) ;
#11880=AXIS2_PLACEMENT_3D ( 'NONE', #1023, #19648, #7759 ) ;
#11884=CIRCLE ( 'NONE', #2046, 7.500000000000007105 ) ;
#11916=EDGE_CURVE ( 'NONE', #15753, #14607, #13306, .T. ) ;
#11931=DIRECTION ( 'NONE',  ( -0.5010362705417042983, 0.000000000000000000, -0.8654262854811264338 ) ) ;
#11939=ORIENTED_EDGE ( 'NONE', *, *, #16049, .T. ) ;
#11940=DIRECTION ( 'NONE',  ( -0.8654262854811262118, 0.000000000000000000, -0.5010362705417046314 ) ) ;
#11945=DIRECTION ( 'NONE',  ( 0.000000000000000000, 0.000000000000000000, -1.000000000000000000 ) ) ;
#11950=AXIS2_PLACEMENT_3D ( 'NONE', #5141, #21793, #10220 ) ;
#11988=DIRECTION ( 'NONE',  ( 1.186952418100008983E-16, 0.000000000000000000, 1.000000000000000000 ) ) ;
#11995=DIRECTION ( 'NONE',  ( -0.000000000000000000, 0.000000000000000000, 1.000000000000000000 ) ) ;
#12027=VERTEX_POINT ( 'NONE', #15035 ) ;
#12032=ORIENTED_EDGE ( 'NONE', *, *, #17944, .F. ) ;
#12036=DIRECTION ( 'NONE',  ( 0.000000000000000000, -1.000000000000000000, 0.000000000000000000 ) ) ;
#12037=EDGE_CURVE ( 'NONE', #4573, #18529, #9788, .T. ) ;
#12043=ORIENTED_EDGE ( 'NONE', *, *, #12037, .T. ) ;
#12045=FACE_OUTER_BOUND ( 'NONE', #20267, .T. ) ;
#12053=EDGE_CURVE ( 'NONE', #21314, #15790, #19783, .T. ) ;
#12060=EDGE_LOOP ( 'NONE', ( #6122, #17849 ) ) ;
#12100=CYLINDRICAL_SURFACE ( 'NONE', #16343, 10.00000000000000888 ) ;
#12101=( LENGTH_UNIT ( ) NAMED_UNIT ( * ) SI_UNIT ( .MILLI., .METRE. ) );
#12137=CARTESIAN_POINT ( 'NONE',  ( -151.4692556286852891, -126.9891397928655010, 39.65701158161630246 ) ) ;
#12142=ORIENTED_EDGE ( 'NONE', *, *, #15076, .T. ) ;
#12147=EDGE_CURVE ( 'NONE', #4877, #10397, #5207, .T. ) ;
#12151=CARTESIAN_POINT ( 'NONE',  ( -39.63192160874135084, -354.7018910364275257, 20.00000000000002132 ) ) ;
#12154=EDGE_CURVE ( 'NONE', #14607, #15753, #18226, .T. ) ;
#12200=EDGE_CURVE ( 'NONE', #10861, #1573, #11884, .T. ) ;
#12212=FACE_BOUND ( 'NONE', #1636, .T. ) ;
#12213=LINE ( 'NONE', #15315, #5503 ) ;
#12221=LINE ( 'NONE', #2092, #68 ) ;
#12231=ORIENTED_EDGE ( 'NONE', *, *, #15022, .T. ) ;
#12266=DIRECTION ( 'NONE',  ( 0.000000000000000000, 0.000000000000000000, -1.000000000000000000 ) ) ;
#12297=ORIENTED_EDGE ( 'NONE', *, *, #12053, .T. ) ;
#12319=DIRECTION ( 'NONE',  ( 0.000000000000000000, -0.000000000000000000, -1.000000000000000000 ) ) ;
#12330=PLANE ( 'NONE',  #10243 ) ;
#12332=EDGE_CURVE ( 'NONE', #5667, #10538, #15477, .T. ) ;
#12344=CARTESIAN_POINT ( 'NONE',  ( 126.8576204525573274, -126.9891397928655010, 67.64809332337412684 ) ) ;
#12352=CARTESIAN_POINT ( 'NONE',  ( 43.01140435219951996, 119.9070776186055838, -35.00000000000000000 ) ) ;
#12358=FACE_BOUND ( 'NONE', #12466, .T. ) ;
#12363=VERTEX_POINT ( 'NONE', #4320 ) ;
#12375=VECTOR ( 'NONE', #270, 1000.000000000000000 ) ;
#12386=EDGE_LOOP ( 'NONE', ( #18338, #12705, #3674, #16726, #10238, #9940, #18221, #1807, #6721, #7252 ) ) ;
#12412=ORIENTED_EDGE ( 'NONE', *, *, #601, .T. ) ;
#12421=ORIENTED_EDGE ( 'NONE', *, *, #929, .F. ) ;
#12466=EDGE_LOOP ( 'NONE', ( #3240, #14980 ) ) ;
#12468=EDGE_CURVE ( 'NONE', #4975, #5215, #5533, .T. ) ;
#12471=ORIENTED_EDGE ( 'NONE', *, *, #18144, .T. ) ;
#12475=CIRCLE ( 'NONE', #11766, 10.00000000000000888 ) ;
#12476=DIRECTION ( 'NONE',  ( 1.000000000000000000, -0.000000000000000000, -1.140132994654635861E-16 ) ) ;
#12489=ORIENTED_EDGE ( 'NONE', *, *, #21126, .F. ) ;
#12503=ORIENTED_EDGE ( 'NONE', *, *, #8140, .T. ) ;
#12565=DIRECTION ( 'NONE',  ( 0.000000000000000000, 0.000000000000000000, 1.000000000000000000 ) ) ;
#12583=ORIENTED_EDGE ( 'NONE', *, *, #11250, .F. ) ;
#12584=EDGE_CURVE ( 'NONE', #13613, #13351, #6840, .T. ) ;
#12587=EDGE_CURVE ( 'NONE', #11679, #2742, #20690, .T. ) ;
#12590=CARTESIAN_POINT ( 'NONE',  ( 116.4417310231185780, -136.9891397928655010, 0.3429884183836981459 ) ) ;
#12611=LINE ( 'NONE', #19333, #7296 ) ;
#12638=ORIENTED_EDGE ( 'NONE', *, *, #16551, .T. ) ;
#12641=AXIS2_PLACEMENT_3D ( 'NONE', #11553, #2957, #19945 ) ;
#12657=AXIS2_PLACEMENT_3D ( 'NONE', #2403, #7050, #17169 ) ;
#12661=CARTESIAN_POINT ( 'NONE',  ( 0.000000000000000000, 160.7104996726487514, -25.00000000000000000 ) ) ;
#12663=ORIENTED_EDGE ( 'NONE', *, *, #7587, .T. ) ;
#12678=FACE_OUTER_BOUND ( 'NONE', #3408, .T. ) ;
#12681=VERTEX_POINT ( 'NONE', #16741 ) ;
#12683=VERTEX_POINT ( 'NONE', #11450 ) ;
#12705=ORIENTED_EDGE ( 'NONE', *, *, #11834, .T. ) ;
#12711=ORIENTED_EDGE ( 'NONE', *, *, #13822, .T. ) ;
#12716=ORIENTED_EDGE ( 'NONE', *, *, #3684, .F. ) ;
#12718=ORIENTED_EDGE ( 'NONE', *, *, #10314, .F. ) ;
#12730=AXIS2_PLACEMENT_3D ( 'NONE', #1510, #18259, #17916 ) ;
#12731=ADVANCED_FACE ( 'NONE', ( #19942, #15192, #19824, #16835 ), #20269, .T. ) ;
#12744=AXIS2_PLACEMENT_3D ( 'NONE', #13925, #2143, #10529 ) ;
#12769=VERTEX_POINT ( 'NONE', #20167 ) ;
#12779=DIRECTION ( 'NONE',  ( 1.000000000000000000, 0.000000000000000000, 0.000000000000000000 ) ) ;
#12813=VERTEX_POINT ( 'NONE', #16500 ) ;
#12824=AXIS2_PLACEMENT_3D ( 'NONE', #2294, #2089, #17281 ) ;
#12845=ORIENTED_EDGE ( 'NONE', *, *, #14009, .F. ) ;
#12864=FACE_BOUND ( 'NONE', #16533, .T. ) ;
#12873=CARTESIAN_POINT ( 'NONE',  ( 126.8576204525573274, -136.9891397928655010, -17.64809332337413750 ) ) ;
#12879=EDGE_CURVE ( 'NONE', #4859, #16995, #14152, .T. ) ;
#12880=ORIENTED_EDGE ( 'NONE', *, *, #10439, .T. ) ;
#12882=ORIENTED_EDGE ( 'NONE', *, *, #15389, .T. ) ;
#12898=CARTESIAN_POINT ( 'NONE',  ( -151.4692556286852891, -126.9891397928655010, -44.65701158161626694 ) ) ;
#12911=ORIENTED_EDGE ( 'NONE', *, *, #16291, .T. ) ;
#12912=ORIENTED_EDGE ( 'NONE', *, *, #8265, .T. ) ;
#12922=VECTOR ( 'NONE', #7617, 1000.000000000000000 ) ;
#12935=VECTOR ( 'NONE', #20240, 1000.000000000000000 ) ;
#12938=EDGE_LOOP ( 'NONE', ( #18209, #4547, #19015, #3009 ) ) ;
#12945=CARTESIAN_POINT ( 'NONE',  ( -176.9699209214867892, 482.8605407899846682, -19.99999999999995737 ) ) ;
#12949=DIRECTION ( 'NONE',  ( 1.000000000000000000, 0.000000000000000000, 0.000000000000000000 ) ) ;
#12957=CARTESIAN_POINT ( 'NONE',  ( 18.67254549292281141, -61.68114226949890622, 30.00000000000000000 ) ) ;
#12965=ORIENTED_EDGE ( 'NONE', *, *, #21126, .T. ) ;
#13068=DIRECTION ( 'NONE',  ( 1.140132994654635861E-16, 0.000000000000000000, 1.000000000000000000 ) ) ;
#13094=PLANE ( 'NONE',  #4286 ) ;
#13098=EDGE_LOOP ( 'NONE', ( #6578, #2456 ) ) ;
#13112=CARTESIAN_POINT ( 'NONE',  ( -46.09493621325655255, 160.7104996726487229, -25.00000000000000000 ) ) ;
#13129=ORIENTED_EDGE ( 'NONE', *, *, #4244, .F. ) ;
#13138=CYLINDRICAL_SURFACE ( 'NONE', #19917, 7.500000000000007105 ) ;
#13142=DIRECTION ( 'NONE',  ( 0.000000000000000000, 0.000000000000000000, 1.000000000000000000 ) ) ;
#13150=CARTESIAN_POINT ( 'NONE',  ( 173.3794444120442506, -136.9891397928655010, 67.64809332337412684 ) ) ;
#13181=ORIENTED_EDGE ( 'NONE', *, *, #17540, .F. ) ;
#13226=VECTOR ( 'NONE', #13598, 1000.000000000000000 ) ;
#13237=ORIENTED_EDGE ( 'NONE', *, *, #16049, .F. ) ;
#13239=CARTESIAN_POINT ( 'NONE',  ( -151.4692556286852891, -136.9891397928655010, -44.65701158161626694 ) ) ;
#13243=VECTOR ( 'NONE', #1139, 1000.000000000000000 ) ;
#13250=DIRECTION ( 'NONE',  ( 0.000000000000000000, 0.000000000000000000, 1.000000000000000000 ) ) ;
#13255=ORIENTED_EDGE ( 'NONE', *, *, #13552, .F. ) ;
#13289=CIRCLE ( 'NONE', #11880, 27.58651506682278765 ) ;
#13296=PRODUCT ( 'Cast Steel Heavy Body Block', 'Cast Steel Heavy Body Block', '', ( #14920 ) ) ;
#13298=EDGE_LOOP ( 'NONE', ( #13792, #15391, #10638, #4947 ) ) ;
#13306=CIRCLE ( 'NONE', #7688, 10.00000000000000888 ) ;
#13316=DIRECTION ( 'NONE',  ( -0.000000000000000000, -0.000000000000000000, 1.000000000000000000 ) ) ;
#13351=VERTEX_POINT ( 'NONE', #3677 ) ;
#13365=EDGE_CURVE ( 'NONE', #13351, #14655, #2334, .T. ) ;
#13387=CARTESIAN_POINT ( 'NONE',  ( -130.4480969619998234, -126.9891397928655010, 67.64809332337415526 ) ) ;
#13397=DIRECTION ( 'NONE',  ( 1.000000000000000000, 0.000000000000000000, 0.000000000000000000 ) ) ;
#13408=CARTESIAN_POINT ( 'NONE',  ( 83.67254549292280785, -61.68114226949890622, -46.21320343559645494 ) ) ;
#13428=EDGE_CURVE ( 'NONE', #7232, #17291, #2675, .T. ) ;
#13429=CARTESIAN_POINT ( 'NONE',  ( 0.000000000000000000, 0.000000000000000000, 30.00000000000000000 ) ) ;
#13430=VERTEX_POINT ( 'NONE', #11718 ) ;
#13439=DIRECTION ( 'NONE',  ( -1.000000000000000000, 0.000000000000000000, -5.966140889015784385E-16 ) ) ;
#13442=CARTESIAN_POINT ( 'NONE',  ( -151.4692556286852891, -126.9891397928655010, 49.65701158161630957 ) ) ;
#13457=ORIENTED_EDGE ( 'NONE', *, *, #16105, .F. ) ;
#13458=EDGE_LOOP ( 'NONE', ( #8144, #13457, #9394, #1171 ) ) ;
#13468=FACE_OUTER_BOUND ( 'NONE', #16119, .T. ) ;
#13509=EDGE_CURVE ( 'NONE', #13722, #12813, #11489, .T. ) ;
#13517=DIRECTION ( 'NONE',  ( 1.000000000000000000, 0.000000000000000000, 0.000000000000000000 ) ) ;
#13520=DIRECTION ( 'NONE',  ( 0.000000000000000000, -1.000000000000000000, 0.000000000000000000 ) ) ;
#13542=CARTESIAN_POINT ( 'NONE',  ( 147.8787791192428074, -126.9891397928655010, 59.65701158161630957 ) ) ;
#13552=EDGE_CURVE ( 'NONE', #18638, #9201, #4104, .T. ) ;
#13568=CARTESIAN_POINT ( 'NONE',  ( 173.3794444120442506, -126.9891397928655010, -17.64809332337413750 ) ) ;
#13573=EDGE_CURVE ( 'NONE', #11274, #784, #10516, .T. ) ;
#13597=DIRECTION ( 'NONE',  ( 1.000000000000000000, 0.000000000000000000, 0.000000000000000000 ) ) ;
#13598=DIRECTION ( 'NONE',  ( 0.000000000000000000, 0.000000000000000000, -1.000000000000000000 ) ) ;
#13600=VECTOR ( 'NONE', #17877, 1000.000000000000000 ) ;
#13613=VERTEX_POINT ( 'NONE', #18994 ) ;
#13614=VECTOR ( 'NONE', #21611, 1000.000000000000000 ) ;
#13628=AXIS2_PLACEMENT_3D ( 'NONE', #3920, #10867, #17352 ) ;
#13652=CARTESIAN_POINT ( 'NONE',  ( 116.9721770337685740, 160.7104996726487514, -25.00000000000000000 ) ) ;
#13658=CARTESIAN_POINT ( 'NONE',  ( 173.3794444120442506, 0.000000000000000000, 30.00000000000000000 ) ) ;
#13663=EDGE_CURVE ( 'NONE', #16995, #12027, #10727, .T. ) ;
#13666=ORIENTED_EDGE ( 'NONE', *, *, #12147, .F. ) ;
#13671=DIRECTION ( 'NONE',  ( -0.5010362705417045204, -0.000000000000000000, 0.8654262854811263228 ) ) ;
#13676=CARTESIAN_POINT ( 'NONE',  ( 147.8787791192428074, -126.9891397928655010, 59.65701158161630957 ) ) ;
#13683=CARTESIAN_POINT ( 'NONE',  ( 147.8787791192428074, -136.9891397928655010, 39.65701158161628825 ) ) ;
#13722=VERTEX_POINT ( 'NONE', #16104 ) ;
#13728=LINE ( 'NONE', #16401, #4560 ) ;
#13739=FACE_OUTER_BOUND ( 'NONE', #11686, .T. ) ;
#13782=CARTESIAN_POINT ( 'NONE',  ( 111.4021762516569964, 137.5714195593754710, -19.99999999999997868 ) ) ;
#13792=ORIENTED_EDGE ( 'NONE', *, *, #20803, .F. ) ;
#13821=ORIENTED_EDGE ( 'NONE', *, *, #9831, .F. ) ;
#13822=EDGE_CURVE ( 'NONE', #1116, #12681, #17753, .T. ) ;
#13825=LINE ( 'NONE', #2042, #14135 ) ;
#13830=ORIENTED_EDGE ( 'NONE', *, *, #12584, .F. ) ;
#13840=CARTESIAN_POINT ( 'NONE',  ( 173.3794444120442506, -136.9891397928655010, -17.64809332337413750 ) ) ;
#13862=CARTESIAN_POINT ( 'NONE',  ( 116.4417310231185780, -126.9891397928655010, 49.65701158161629536 ) ) ;
#13872=CARTESIAN_POINT ( 'NONE',  ( 116.9721770337685740, 160.7104996726487798, -19.99999999999999289 ) ) ;
#13873=AXIS2_PLACEMENT_3D ( 'NONE', #8815, #5592, #12319 ) ;
#13886=AXIS2_PLACEMENT_3D ( 'NONE', #5808, #4478, #9350 ) ;
#13890=DIRECTION ( 'NONE',  ( 1.000000000000000000, 0.000000000000000000, 0.000000000000000000 ) ) ;
#13901=CARTESIAN_POINT ( 'NONE',  ( -130.4480969619997950, -126.9891397928655010, -72.64809332337412684 ) ) ;
#13917=CARTESIAN_POINT ( 'NONE',  ( -47.86331837773882825, -37.13255853780189852, -19.99999999999997158 ) ) ;
#13925=CARTESIAN_POINT ( 'NONE',  ( -151.4692556286852891, -126.9891397928655010, -54.65701158161630246 ) ) ;
#13938=DIRECTION ( 'NONE',  ( 1.000000000000000000, 0.000000000000000000, -2.229410185538112728E-16 ) ) ;
#13943=DIRECTION ( 'NONE',  ( -0.000000000000000000, -0.000000000000000000, 1.000000000000000000 ) ) ;
#13952=ORIENTED_EDGE ( 'NONE', *, *, #8265, .F. ) ;
#13969=PLANE ( 'NONE',  #7210 ) ;
#13971=PLANE ( 'NONE',  #13873 ) ;
#13986=AXIS2_PLACEMENT_3D ( 'NONE', #9297, #803, #9083 ) ;
#13999=AXIS2_PLACEMENT_3D ( 'NONE', #12957, #21783, #13397 ) ;
#14009=EDGE_CURVE ( 'NONE', #18451, #40, #6965, .T. ) ;
#14017=ORIENTED_EDGE ( 'NONE', *, *, #9609, .T. ) ;
#14024=DIRECTION ( 'NONE',  ( -1.000000000000000000, 0.000000000000000000, -1.233581138472395521E-15 ) ) ;
#14028=DIRECTION ( 'NONE',  ( 0.000000000000000000, 0.000000000000000000, -1.000000000000000000 ) ) ;
#14043=DIRECTION ( 'NONE',  ( 1.000000000000000000, 0.000000000000000000, 0.000000000000000000 ) ) ;
#14055=CARTESIAN_POINT ( 'NONE',  ( 18.67254549292281141, -61.68114226949890622, 20.00000000000000355 ) ) ;
#14105=CARTESIAN_POINT ( 'NONE',  ( -32.30114424549768870, -19.06233958201669410, -25.00000000000000000 ) ) ;
#14119=ORIENTED_EDGE ( 'NONE', *, *, #10481, .T. ) ;
#14135=VECTOR ( 'NONE', #7339, 1000.000000000000114 ) ;
#14142=VECTOR ( 'NONE', #4026, 1000.000000000000000 ) ;
#14152=LINE ( 'NONE', #9212, #6978 ) ;
#14153=VECTOR ( 'NONE', #20554, 1000.000000000000000 ) ;
#14187=( NAMED_UNIT ( * ) SI_UNIT ( $, .STERADIAN. ) SOLID_ANGLE_UNIT ( ) );
#14193=CARTESIAN_POINT ( 'NONE',  ( 132.3486983259487886, 110.2203079035326851, -35.00000000000000000 ) ) ;
#14200=DIRECTION ( 'NONE',  ( 0.000000000000000000, -1.000000000000000000, 0.000000000000000000 ) ) ;
#14211=CYLINDRICAL_SURFACE ( 'NONE', #17086, 15.56217413224114310 ) ;
#14212=ADVANCED_FACE ( 'NONE', ( #19016 ), #7343, .T. ) ;
#14231=AXIS2_PLACEMENT_3D ( 'NONE', #3786, #11940, #10405 ) ;
#14251=CIRCLE ( 'NONE', #8645, 7.500000000000000000 ) ;
#14257=EDGE_CURVE ( 'NONE', #20193, #12027, #12611, .T. ) ;
#14262=LINE ( 'NONE', #4138, #261 ) ;
#14280=( GEOMETRIC_REPRESENTATION_CONTEXT ( 3 ) GLOBAL_UNCERTAINTY_ASSIGNED_CONTEXT ( ( #5758 ) ) GLOBAL_UNIT_ASSIGNED_CONTEXT ( ( #9575, #14411, #863 ) ) REPRESENTATION_CONTEXT ( 'NONE', 'WORKASPACE' ) );
#14302=CARTESIAN_POINT ( 'NONE',  ( 173.3794444120442506, 0.000000000000000000, 30.00000000000000000 ) ) ;
#14310=LINE ( 'NONE', #8764, #14153 ) ;
#14342=VERTEX_POINT ( 'NONE', #4021 ) ;
#14344=CARTESIAN_POINT ( 'NONE',  ( 43.01140435219951996, 119.9070776186055838, -19.99999999999997868 ) ) ;
#14360=ORIENTED_EDGE ( 'NONE', *, *, #601, .F. ) ;
#14376=DIRECTION ( 'NONE',  ( -0.000000000000000000, -0.000000000000000000, -1.000000000000000000 ) ) ;
#14394=ORIENTED_EDGE ( 'NONE', *, *, #9609, .F. ) ;
#14396=AXIS2_PLACEMENT_3D ( 'NONE', #6829, #7477, #4051 ) ;
#14411=( NAMED_UNIT ( * ) PLANE_ANGLE_UNIT ( ) SI_UNIT ( $, .RADIAN. ) );
#14415=DIRECTION ( 'NONE',  ( 1.000000000000000000, 0.000000000000000000, 0.000000000000000000 ) ) ;
#14417=DIRECTION ( 'NONE',  ( 0.000000000000000000, 0.000000000000000000, 1.000000000000000000 ) ) ;
#14421=ORIENTED_EDGE ( 'NONE', *, *, #4976, .T. ) ;
#14423=CARTESIAN_POINT ( 'NONE',  ( -151.4692556286852891, -126.9891397928655010, -54.65701158161630246 ) ) ;
#14465=LINE ( 'NONE', #13150, #1979 ) ;
#14471=ORIENTED_EDGE ( 'NONE', *, *, #1773, .T. ) ;
#14475=VECTOR ( 'NONE', #1408, 1000.000000000000000 ) ;
#14478=DIRECTION ( 'NONE',  ( 1.000000000000000000, 0.000000000000000000, 0.000000000000000000 ) ) ;
#14479=LINE ( 'NONE', #2580, #2800 ) ;
#14493=CARTESIAN_POINT ( 'NONE',  ( 141.1725454929228079, -61.68114226949890622, -46.21320343559645494 ) ) ;
#14494=ORIENTED_EDGE ( 'NONE', *, *, #16312, .F. ) ;
#14503=LINE ( 'NONE', #9239, #16790 ) ;
#14504=CIRCLE ( 'NONE', #17320, 7.500000000000007105 ) ;
#14514=FACE_BOUND ( 'NONE', #15024, .T. ) ;
#14519=PRESENTATION_STYLE_ASSIGNMENT (( #5926 ) ) ;
#14528=ORIENTED_EDGE ( 'NONE', *, *, #19865, .T. ) ;
#14536=CARTESIAN_POINT ( 'NONE',  ( 173.3794444120442506, -126.9891397928655010, -17.64809332337413750 ) ) ;
#14564=CARTESIAN_POINT ( 'NONE',  ( 144.5586921005913439, 160.7104996726487798, -19.99999999999999645 ) ) ;
#14575=CIRCLE ( 'NONE', #850, 15.56217413224114310 ) ;
#14577=ORIENTED_EDGE ( 'NONE', *, *, #6191, .T. ) ;
#14579=ORIENTED_EDGE ( 'NONE', *, *, #17944, .T. ) ;
#14602=DIRECTION ( 'NONE',  ( 1.000000000000000000, 0.000000000000000000, -1.140132994654635861E-16 ) ) ;
#14606=ORIENTED_EDGE ( 'NONE', *, *, #9756, .F. ) ;
#14607=VERTEX_POINT ( 'NONE', #18424 ) ;
#14611=CIRCLE ( 'NONE', #1601, 10.00000000000000888 ) ;
#14625=DIRECTION ( 'NONE',  ( -0.000000000000000000, -0.000000000000000000, 1.000000000000000000 ) ) ;
#14642=CARTESIAN_POINT ( 'NONE',  ( 18.67254549292281141, -61.68114226949890622, -46.21320343559645494 ) ) ;
#14647=DIRECTION ( 'NONE',  ( -1.000000000000000000, -0.000000000000000000, -0.000000000000000000 ) ) ;
#14655=VERTEX_POINT ( 'NONE', #13239 ) ;
#14677=AXIS2_PLACEMENT_3D ( 'NONE', #14642, #2853, #12779 ) ;
#14694=AXIS2_PLACEMENT_3D ( 'NONE', #5232, #10306, #7216 ) ;
#14717=ADVANCED_FACE ( 'NONE', ( #17290 ), #7502, .T. ) ;
#14746=VERTEX_POINT ( 'NONE', #15439 ) ;
#14783=PLANE ( 'NONE',  #4417 ) ;
#14787=CARTESIAN_POINT ( 'NONE',  ( -120.0322075325610598, -136.9891397928655010, -54.65701158161630246 ) ) ;
#14801=ORIENTED_EDGE ( 'NONE', *, *, #3391, .F. ) ;
#14807=LINE ( 'NONE', #12945, #7491 ) ;
#14823=VERTEX_POINT ( 'NONE', #17183 ) ;
#14840=VECTOR ( 'NONE', #14625, 1000.000000000000000 ) ;
#14843=LINE ( 'NONE', #12873, #21407 ) ;
#14868=ADVANCED_FACE ( 'NONE', ( #3648 ), #8934, .T. ) ;
#14892=DIRECTION ( 'NONE',  ( 0.000000000000000000, -1.000000000000000000, 0.000000000000000000 ) ) ;
#14920=PRODUCT_CONTEXT ( 'NONE', #19855, 'mechanical' ) ;
#14938=VECTOR ( 'NONE', #3275, 1000.000000000000000 ) ;
#14968=DIRECTION ( 'NONE',  ( 0.000000000000000000, -1.000000000000000000, 0.000000000000000000 ) ) ;
#14977=CIRCLE ( 'NONE', #3014, 10.00000000000000888 ) ;
#14980=ORIENTED_EDGE ( 'NONE', *, *, #20278, .T. ) ;
#14990=ORIENTED_EDGE ( 'NONE', *, *, #7982, .T. ) ;
#14991=EDGE_CURVE ( 'NONE', #18069, #8286, #11329, .T. ) ;
#15021=ORIENTED_EDGE ( 'NONE', *, *, #20781, .F. ) ;
#15022=EDGE_CURVE ( 'NONE', #4009, #20322, #4279, .T. ) ;
#15024=EDGE_LOOP ( 'NONE', ( #4205, #18108 ) ) ;
#15026=CARTESIAN_POINT ( 'NONE',  ( -151.4692556286852891, -126.9891397928655010, 49.65701158161630957 ) ) ;
#15033=DIRECTION ( 'NONE',  ( 0.000000000000000000, 0.000000000000000000, 1.000000000000000000 ) ) ;
#15035=CARTESIAN_POINT ( 'NONE',  ( 173.3794444120442222, -37.13255853780189852, 19.99999999999999645 ) ) ;
#15051=EDGE_LOOP ( 'NONE', ( #20539, #17718 ) ) ;
#15053=APPLICATION_CONTEXT ( 'automotive_design' ) ;
#15076=EDGE_CURVE ( 'NONE', #8286, #13722, #2954, .T. ) ;
#15087=DIRECTION ( 'NONE',  ( 0.000000000000000000, -1.000000000000000000, 0.000000000000000000 ) ) ;
#15108=ORIENTED_EDGE ( 'NONE', *, *, #19413, .T. ) ;
#15111=CIRCLE ( 'NONE', #8072, 7.500000000000000000 ) ;
#15117=DIRECTION ( 'NONE',  ( -1.000000000000000000, -0.000000000000000000, -0.000000000000000000 ) ) ;
#15121=CARTESIAN_POINT ( 'NONE',  ( -176.9699209214867892, -37.13255853780189852, 30.00000000000000000 ) ) ;
#15126=EDGE_CURVE ( 'NONE', #8531, #15585, #14310, .T. ) ;
#15144=CARTESIAN_POINT ( 'NONE',  ( 53.01140435219953417, 119.9070776186055838, -35.00000000000000000 ) ) ;
#15146=CARTESIAN_POINT ( 'NONE',  ( -151.4692556286852891, -136.9891397928655010, 49.65701158161630957 ) ) ;
#15168=EDGE_CURVE ( 'NONE', #8458, #19770, #5336, .T. ) ;
#15183=CYLINDRICAL_SURFACE ( 'NONE', #15760, 10.00000000000000888 ) ;
#15191=ORIENTED_EDGE ( 'NONE', *, *, #13509, .T. ) ;
#15192=FACE_BOUND ( 'NONE', #2932, .T. ) ;
#15204=VECTOR ( 'NONE', #10906, 1000.000000000000114 ) ;
#15211=AXIS2_PLACEMENT_3D ( 'NONE', #17243, #4134, #17459 ) ;
#15260=DIRECTION ( 'NONE',  ( 0.000000000000000000, 0.000000000000000000, 1.000000000000000000 ) ) ;
#15277=VERTEX_POINT ( 'NONE', #19427 ) ;
#15280=LINE ( 'NONE', #18477, #16497 ) ;
#15281=EDGE_CURVE ( 'NONE', #4552, #15878, #805, .T. ) ;
#15287=FACE_OUTER_BOUND ( 'NONE', #13298, .T. ) ;
#15315=CARTESIAN_POINT ( 'NONE',  ( -39.63192160874135084, -136.9891397928655010, 20.00000000000002132 ) ) ;
#15341=VECTOR ( 'NONE', #3873, 1000.000000000000000 ) ;
#15384=ORIENTED_EDGE ( 'NONE', *, *, #9526, .T. ) ;
#15389=EDGE_CURVE ( 'NONE', #14823, #6453, #15789, .T. ) ;
#15391=ORIENTED_EDGE ( 'NONE', *, *, #2276, .F. ) ;
#15398=LINE ( 'NONE', #2160, #3436 ) ;
#15405=AXIS2_PLACEMENT_3D ( 'NONE', #7679, #5781, #6106 ) ;
#15411=CARTESIAN_POINT ( 'NONE',  ( -120.0322075325610740, -126.9891397928655010, 30.00000000000000000 ) ) ;
#15437=EDGE_LOOP ( 'NONE', ( #17829, #19510, #17483, #7974 ) ) ;
#15439=CARTESIAN_POINT ( 'NONE',  ( 116.4417310231185780, -126.9891397928655010, 30.00000000000000000 ) ) ;
#15468=ORIENTED_EDGE ( 'NONE', *, *, #3630, .F. ) ;
#15477=LINE ( 'NONE', #19001, #285 ) ;
#15493=ORIENTED_EDGE ( 'NONE', *, *, #2798, .F. ) ;
#15510=CARTESIAN_POINT ( 'NONE',  ( 43.01140435219951996, 119.9070776186055838, -35.00000000000000000 ) ) ;
#15524=DIRECTION ( 'NONE',  ( 1.000000000000000000, 0.000000000000000000, 0.000000000000000000 ) ) ;
#15554=CARTESIAN_POINT ( 'NONE',  ( -176.9699209214867608, -126.9891397928655010, 30.00000000000000000 ) ) ;
#15585=VERTEX_POINT ( 'NONE', #1131 ) ;
#15590=ORIENTED_EDGE ( 'NONE', *, *, #15168, .F. ) ;
#15601=AXIS2_PLACEMENT_3D ( 'NONE', #20306, #14892, #13250 ) ;
#15622=DIRECTION ( 'NONE',  ( 0.000000000000000000, -1.000000000000000000, 0.000000000000000000 ) ) ;
#15623=DIRECTION ( 'NONE',  ( -0.000000000000000000, -0.000000000000000000, 1.000000000000000000 ) ) ;
#15631=FACE_BOUND ( 'NONE', #12060, .T. ) ;
#15637=DIRECTION ( 'NONE',  ( 0.000000000000000000, -0.000000000000000000, -1.000000000000000000 ) ) ;
#15658=ORIENTED_EDGE ( 'NONE', *, *, #19345, .T. ) ;
#15673=VECTOR ( 'NONE', #2479, 1000.000000000000000 ) ;
#15681=DIRECTION ( 'NONE',  ( 0.000000000000000000, -1.000000000000000000, 0.000000000000000000 ) ) ;
#15683=ORIENTED_EDGE ( 'NONE', *, *, #13428, .T. ) ;
#15699=ORIENTED_EDGE ( 'NONE', *, *, #11424, .T. ) ;
#15704=LINE ( 'NONE', #2157, #1836 ) ;
#15735=VECTOR ( 'NONE', #1149, 1000.000000000000000 ) ;
#15751=AXIS2_PLACEMENT_3D ( 'NONE', #21094, #15681, #14028 ) ;
#15753=VERTEX_POINT ( 'NONE', #13683 ) ;
#15760=AXIS2_PLACEMENT_3D ( 'NONE', #15510, #1741, #16933 ) ;
#15789=LINE ( 'NONE', #5760, #16950 ) ;
#15790=VERTEX_POINT ( 'NONE', #20417 ) ;
#15801=ORIENTED_EDGE ( 'NONE', *, *, #2549, .T. ) ;
#15812=DIRECTION ( 'NONE',  ( 1.000000000000000000, 0.000000000000000000, 0.000000000000000000 ) ) ;
#15820=ORIENTED_EDGE ( 'NONE', *, *, #6558, .T. ) ;
#15850=PLANE ( 'NONE',  #1794 ) ;
#15853=EDGE_CURVE ( 'NONE', #10538, #119, #11701, .T. ) ;
#15854=CIRCLE ( 'NONE', #6359, 10.00000000000000888 ) ;
#15867=DIRECTION ( 'NONE',  ( -0.000000000000000000, -0.000000000000000000, 1.000000000000000000 ) ) ;
#15878=VERTEX_POINT ( 'NONE', #18653 ) ;
#15920=DIRECTION ( 'NONE',  ( 0.000000000000000000, -1.000000000000000000, 0.000000000000000000 ) ) ;
#15939=CARTESIAN_POINT ( 'NONE',  ( -46.09493621325655255, 160.7104996726487798, -19.99999999999997158 ) ) ;
#15947=LINE ( 'NONE', #11100, #21635 ) ;
#15955=DIRECTION ( 'NONE',  ( -1.000000000000000000, 0.000000000000000000, 0.000000000000000000 ) ) ;
#15959=ADVANCED_FACE ( 'NONE', ( #559 ), #5843, .F. ) ;
#15979=EDGE_LOOP ( 'NONE', ( #6850, #16148, #15820, #16646 ) ) ;
#15990=AXIS2_PLACEMENT_3D ( 'NONE', #10333, #18598, #20362 ) ;
#16031=EDGE_LOOP ( 'NONE', ( #11248, #278, #12912, #6867 ) ) ;
#16044=AXIS2_PLACEMENT_3D ( 'NONE', #1680, #11592, #8079 ) ;
#16046=ADVANCED_FACE ( 'NONE', ( #3059 ), #7814, .T. ) ;
#16049=EDGE_CURVE ( 'NONE', #735, #18451, #17927, .T. ) ;
#16053=PLANE ( 'NONE',  #13886 ) ;
#16063=CARTESIAN_POINT ( 'NONE',  ( 43.01140435219951996, 119.9070776186055838, -19.99999999999997868 ) ) ;
#16072=VECTOR ( 'NONE', #15087, 1000.000000000000000 ) ;
#16079=CARTESIAN_POINT ( 'NONE',  ( -9.888205435155610346, 14.72870593739803624, -19.99999999999997868 ) ) ;
#16103=AXIS2_PLACEMENT_3D ( 'NONE', #11517, #13068, #14602 ) ;
#16104=CARTESIAN_POINT ( 'NONE',  ( 33.01140435219951286, 119.9070776186055838, -19.99999999999997868 ) ) ;
#16105=EDGE_CURVE ( 'NONE', #13613, #4745, #3598, .T. ) ;
#16119=EDGE_LOOP ( 'NONE', ( #11654, #14528, #15699, #9260 ) ) ;
#16124=ORIENTED_EDGE ( 'NONE', *, *, #11768, .F. ) ;
#16128=ORIENTED_EDGE ( 'NONE', *, *, #11356, .T. ) ;
#16134=CARTESIAN_POINT ( 'NONE',  ( -9.888205435155610346, 14.72870593739803624, -35.00000000000000000 ) ) ;
#16135=CARTESIAN_POINT ( 'NONE',  ( 83.67254549292280785, -61.68114226949890622, 20.00000000000000355 ) ) ;
#16139=LINE ( 'NONE', #19342, #11433 ) ;
#16148=ORIENTED_EDGE ( 'NONE', *, *, #1662, .T. ) ;
#16157=DIRECTION ( 'NONE',  ( 0.000000000000000000, -1.000000000000000000, 0.000000000000000000 ) ) ;
#16161=DIRECTION ( 'NONE',  ( 1.000000000000000000, 0.000000000000000000, 0.000000000000000000 ) ) ;
#16165=CARTESIAN_POINT ( 'NONE',  ( 148.6725454929228079, -61.68114226949890622, -46.21320343559645494 ) ) ;
#16178=ORIENTED_EDGE ( 'NONE', *, *, #5263, .F. ) ;
#16197=ORIENTED_EDGE ( 'NONE', *, *, #20907, .T. ) ;
#16222=ORIENTED_EDGE ( 'NONE', *, *, #21681, .T. ) ;
#16257=FACE_BOUND ( 'NONE', #6402, .T. ) ;
#16288=ORIENTED_EDGE ( 'NONE', *, *, #9356, .T. ) ;
#16291=EDGE_CURVE ( 'NONE', #21749, #8531, #19008, .T. ) ;
#16298=FACE_OUTER_BOUND ( 'NONE', #2095, .T. ) ;
#16312=EDGE_CURVE ( 'NONE', #40, #8611, #167, .T. ) ;
#16314=VERTEX_POINT ( 'NONE', #18790 ) ;
#16328=DIRECTION ( 'NONE',  ( 1.000000000000000000, 0.000000000000000000, 0.000000000000000000 ) ) ;
#16338=CARTESIAN_POINT ( 'NONE',  ( 147.8787791192428074, -136.9891397928655010, -9.657011581616311346 ) ) ;
#16341=ORIENTED_EDGE ( 'NONE', *, *, #16551, .F. ) ;
#16343=AXIS2_PLACEMENT_3D ( 'NONE', #8919, #15623, #15524 ) ;
#16352=DIRECTION ( 'NONE',  ( 0.000000000000000000, -1.000000000000000000, 0.000000000000000000 ) ) ;
#16368=ORIENTED_EDGE ( 'NONE', *, *, #7326, .T. ) ;
#16375=CARTESIAN_POINT ( 'NONE',  ( -39.63192160874126557, -136.9891397928655010, -35.00000000000000000 ) ) ;
#16401=CARTESIAN_POINT ( 'NONE',  ( -120.0322075325610598, -126.9891397928655010, -54.65701158161630246 ) ) ;
#16410=VECTOR ( 'NONE', #20648, 1000.000000000000000 ) ;
#16435=DIRECTION ( 'NONE',  ( 1.000000000000000000, 0.000000000000000000, -1.186952418100008983E-16 ) ) ;
#16478=DIRECTION ( 'NONE',  ( 0.000000000000000000, -0.000000000000000000, 1.000000000000000000 ) ) ;
#16491=CARTESIAN_POINT ( 'NONE',  ( -130.4480969619998234, -126.9891397928655010, 67.64809332337415526 ) ) ;
#16497=VECTOR ( 'NONE', #70, 1000.000000000000000 ) ;
#16500=CARTESIAN_POINT ( 'NONE',  ( 53.01140435219953417, 119.9070776186055838, -19.99999999999997868 ) ) ;
#16512=DIRECTION ( 'NONE',  ( 1.000000000000000000, 0.000000000000000000, 0.000000000000000000 ) ) ;
#16514=CARTESIAN_POINT ( 'NONE',  ( 121.4021762516569964, 137.5714195593754710, -19.99999999999997868 ) ) ;
#16521=ORIENTED_EDGE ( 'NONE', *, *, #7326, .F. ) ;
#16533=EDGE_LOOP ( 'NONE', ( #6180, #766 ) ) ;
#16535=DIRECTION ( 'NONE',  ( 0.5010362705417042983, 0.000000000000000000, 0.8654262854811264338 ) ) ;
#16551=EDGE_CURVE ( 'NONE', #20722, #9507, #13825, .T. ) ;
#16559=EDGE_LOOP ( 'NONE', ( #5026, #682 ) ) ;
#16588=PLANE ( 'NONE',  #11950 ) ;
#16592=CARTESIAN_POINT ( 'NONE',  ( 147.8787791192428074, -126.9891397928655010, 39.65701158161628825 ) ) ;
#16594=DIRECTION ( 'NONE',  ( 0.000000000000000000, 0.000000000000000000, 1.000000000000000000 ) ) ;
#16611=FACE_OUTER_BOUND ( 'NONE', #7192, .T. ) ;
#16619=PRODUCT_DEFINITION_SHAPE ( 'NONE', 'NONE',  #17263 ) ;
#16646=ORIENTED_EDGE ( 'NONE', *, *, #9067, .T. ) ;
#16681=DIRECTION ( 'NONE',  ( 0.000000000000000000, -1.000000000000000000, 0.000000000000000000 ) ) ;
#16682=LINE ( 'NONE', #20227, #11687 ) ;
#16704=VECTOR ( 'NONE', #17921, 1000.000000000000000 ) ;
#16707=CARTESIAN_POINT ( 'NONE',  ( -120.0322075325610598, -136.9891397928655010, -34.99999999999999289 ) ) ;
#16717=DIRECTION ( 'NONE',  ( 1.000000000000000000, 0.000000000000000000, 0.000000000000000000 ) ) ;
#16720=CARTESIAN_POINT ( 'NONE',  ( 116.4417310231185780, -126.9891397928655010, 0.3429884183836981459 ) ) ;
#16723=ORIENTED_EDGE ( 'NONE', *, *, #17447, .T. ) ;
#16726=ORIENTED_EDGE ( 'NONE', *, *, #2549, .F. ) ;
#16738=FACE_OUTER_BOUND ( 'NONE', #3041, .T. ) ;
#16741=CARTESIAN_POINT ( 'NONE',  ( -120.0322075325610598, -136.9891397928655010, -54.65701158161630246 ) ) ;
#16776=AXIS2_PLACEMENT_3D ( 'NONE', #7129, #18479, #13517 ) ;
#16784=ORIENTED_EDGE ( 'NONE', *, *, #15853, .F. ) ;
#16790=VECTOR ( 'NONE', #2496, 1000.000000000000000 ) ;
#16795=CARTESIAN_POINT ( 'NONE',  ( 83.67254549292280785, -61.68114226949890622, 30.00000000000000000 ) ) ;
#16819=CARTESIAN_POINT ( 'NONE',  ( -151.4692556286852891, -126.9891397928655010, 49.65701158161630957 ) ) ;
#16827=LINE ( 'NONE', #20051, #7612 ) ;
#16828=FACE_OUTER_BOUND ( 'NONE', #15437, .T. ) ;
#16835=FACE_BOUND ( 'NONE', #20765, .T. ) ;
#16859=EDGE_LOOP ( 'NONE', ( #1143, #15468, #10937, #19409, #6640 ) ) ;
#16878=ORIENTED_EDGE ( 'NONE', *, *, #1668, .T. ) ;
#16885=ADVANCED_FACE ( 'NONE', ( #5986 ), #20992, .F. ) ;
#16886=FACE_OUTER_BOUND ( 'NONE', #21096, .T. ) ;
#16913=CARTESIAN_POINT ( 'NONE',  ( 91.17254549292282206, -61.68114226949890622, -46.21320343559645494 ) ) ;
#16926=CARTESIAN_POINT ( 'NONE',  ( -120.0322075325610740, -136.9891397928655010, 49.65701158161630957 ) ) ;
#16933=DIRECTION ( 'NONE',  ( 1.000000000000000000, 0.000000000000000000, 0.000000000000000000 ) ) ;
#16938=VERTEX_POINT ( 'NONE', #16338 ) ;
#16941=PLANE ( 'NONE',  #14396 ) ;
#16950=VECTOR ( 'NONE', #4113, 1000.000000000000000 ) ;
#16954=DIRECTION ( 'NONE',  ( -1.233581138472395521E-15, 0.000000000000000000, 1.000000000000000000 ) ) ;
#16959=LINE ( 'NONE', #13658, #509 ) ;
#16966=EDGE_LOOP ( 'NONE', ( #3179, #19228, #2145, #9288 ) ) ;
#16982=PRODUCT_DEFINITION_CONTEXT ( 'detailed design', #15053, 'design' ) ;
#16991=ORIENTED_EDGE ( 'NONE', *, *, #18540, .F. ) ;
#16995=VERTEX_POINT ( 'NONE', #1692 ) ;
#17005=LINE ( 'NONE', #18566, #10651 ) ;
#17011=DIRECTION ( 'NONE',  ( 1.000000000000000000, 0.000000000000000000, -0.000000000000000000 ) ) ;
#17025=ORIENTED_EDGE ( 'NONE', *, *, #19413, .F. ) ;
#17032=AXIS2_PLACEMENT_3D ( 'NONE', #13442, #8381, #6837 ) ;
#17042=DIRECTION ( 'NONE',  ( -0.8654262854811262118, 0.000000000000000000, 0.5010362705417048534 ) ) ;
#17070=AXIS2_PLACEMENT_3D ( 'NONE', #7455, #10758, #5782 ) ;
#17075=EDGE_CURVE ( 'NONE', #12683, #19403, #21651, .T. ) ;
#17076=DIRECTION ( 'NONE',  ( -1.000000000000000000, -2.779543948608941985E-16, 0.000000000000000000 ) ) ;
#17086=AXIS2_PLACEMENT_3D ( 'NONE', #14105, #12565, #5732 ) ;
#17117=CARTESIAN_POINT ( 'NONE',  ( 116.4417310231185780, -126.9891397928655010, 0.3429884183836981459 ) ) ;
#17169=DIRECTION ( 'NONE',  ( 1.000000000000000000, 0.000000000000000000, 0.000000000000000000 ) ) ;
#17176=DIRECTION ( 'NONE',  ( 0.000000000000000000, -1.000000000000000000, 0.000000000000000000 ) ) ;
#17182=ORIENTED_EDGE ( 'NONE', *, *, #17559, .T. ) ;
#17183=CARTESIAN_POINT ( 'NONE',  ( -120.0322075325610598, -126.9891397928655010, -34.99999999999999289 ) ) ;
#17194=CARTESIAN_POINT ( 'NONE',  ( -40.97538603781489996, -6.141859983696321912, -35.00000000000000000 ) ) ;
#17201=ORIENTED_EDGE ( 'NONE', *, *, #9756, .T. ) ;
#17243=CARTESIAN_POINT ( 'NONE',  ( 111.4021762516569964, 137.5714195593754710, -19.99999999999997868 ) ) ;
#17263=PRODUCT_DEFINITION ( 'UNKNOWN', '', #20424, #16982 ) ;
#17278=ADVANCED_FACE ( 'NONE', ( #8855 ), #8957, .T. ) ;
#17281=DIRECTION ( 'NONE',  ( 1.000000000000000000, 0.000000000000000000, -1.186952418100008983E-16 ) ) ;
#17287=FACE_BOUND ( 'NONE', #9278, .T. ) ;
#17290=FACE_OUTER_BOUND ( 'NONE', #2563, .T. ) ;
#17291=VERTEX_POINT ( 'NONE', #12137 ) ;
#17309=ORIENTED_EDGE ( 'NONE', *, *, #21498, .F. ) ;
#17320=AXIS2_PLACEMENT_3D ( 'NONE', #16135, #4446, #14478 ) ;
#17352=DIRECTION ( 'NONE',  ( 1.000000000000000000, 0.000000000000000000, 0.000000000000000000 ) ) ;
#17390=ADVANCED_FACE ( 'NONE', ( #12358, #16886 ), #465, .F. ) ;
#17402=ORIENTED_EDGE ( 'NONE', *, *, #18688, .F. ) ;
#17439=ORIENTED_EDGE ( 'NONE', *, *, #13663, .F. ) ;
#17447=EDGE_CURVE ( 'NONE', #784, #1116, #11792, .T. ) ;
#17459=DIRECTION ( 'NONE',  ( 1.000000000000000000, 0.000000000000000000, 0.000000000000000000 ) ) ;
#17483=ORIENTED_EDGE ( 'NONE', *, *, #1543, .T. ) ;
#17540=EDGE_CURVE ( 'NONE', #20108, #12027, #12221, .T. ) ;
#17559=EDGE_CURVE ( 'NONE', #1608, #8611, #17609, .T. ) ;
#17574=CARTESIAN_POINT ( 'NONE',  ( 116.4417310231185780, -126.9891397928655010, 49.65701158161629536 ) ) ;
#17581=CARTESIAN_POINT ( 'NONE',  ( 116.9721770337685740, 133.1239846058259388, -35.00000000000000000 ) ) ;
#17609=LINE ( 'NONE', #19167, #15204 ) ;
#17644=VERTEX_POINT ( 'NONE', #13872 ) ;
#17646=CARTESIAN_POINT ( 'NONE',  ( -176.9699209214867324, -126.9891397928655010, -72.64809332337415526 ) ) ;
#17666=DIRECTION ( 'NONE',  ( 0.000000000000000000, -1.000000000000000000, 0.000000000000000000 ) ) ;
#17670=CARTESIAN_POINT ( 'NONE',  ( -120.0322075325610740, -126.9891397928655010, 49.65701158161630957 ) ) ;
#17690=ORIENTED_EDGE ( 'NONE', *, *, #315, .T. ) ;
#17696=ORIENTED_EDGE ( 'NONE', *, *, #20278, .F. ) ;
#17718=ORIENTED_EDGE ( 'NONE', *, *, #1662, .F. ) ;
#17731=FACE_OUTER_BOUND ( 'NONE', #7085, .T. ) ;
#17733=CARTESIAN_POINT ( 'NONE',  ( -151.4692556286852891, -126.9891397928655010, 49.65701158161630957 ) ) ;
#17738=EDGE_LOOP ( 'NONE', ( #13821, #142, #8935, #8200 ) ) ;
#17750=ORIENTED_EDGE ( 'NONE', *, *, #3313, .T. ) ;
#17753=LINE ( 'NONE', #9834, #5493 ) ;
#17769=LINE ( 'NONE', #11488, #13600 ) ;
#17775=ORIENTED_EDGE ( 'NONE', *, *, #14009, .T. ) ;
#17783=ADVANCED_FACE ( 'NONE', ( #4600 ), #13094, .F. ) ;
#17800=ORIENTED_EDGE ( 'NONE', *, *, #17075, .F. ) ;
#17801=VERTEX_POINT ( 'NONE', #1085 ) ;
#17803=VECTOR ( 'NONE', #13671, 1000.000000000000114 ) ;
#17804=FACE_OUTER_BOUND ( 'NONE', #8180, .T. ) ;
#17817=CIRCLE ( 'NONE', #16776, 10.00000000000000888 ) ;
#17829=ORIENTED_EDGE ( 'NONE', *, *, #15076, .F. ) ;
#17849=ORIENTED_EDGE ( 'NONE', *, *, #13509, .F. ) ;
#17853=AXIS2_PLACEMENT_3D ( 'NONE', #9868, #7998, #12949 ) ;
#17877=DIRECTION ( 'NONE',  ( 0.000000000000000000, -1.000000000000000000, 0.000000000000000000 ) ) ;
#17903=LINE ( 'NONE', #1497, #20003 ) ;
#17916=DIRECTION ( 'NONE',  ( 1.000000000000000000, 0.000000000000000000, 0.000000000000000000 ) ) ;
#17921=DIRECTION ( 'NONE',  ( 1.000000000000000000, -0.000000000000000000, -0.000000000000000000 ) ) ;
#17927=LINE ( 'NONE', #2837, #14840 ) ;
#17933=EDGE_CURVE ( 'NONE', #12813, #13722, #19095, .T. ) ;
#17944=EDGE_CURVE ( 'NONE', #706, #3989, #2839, .T. ) ;
#17976=CARTESIAN_POINT ( 'NONE',  ( -32.30114424549768870, -19.06233958201669410, -35.00000000000000000 ) ) ;
#17991=ORIENTED_EDGE ( 'NONE', *, *, #3564, .T. ) ;
#18021=ADVANCED_FACE ( 'NONE', ( #5230 ), #1913, .F. ) ;
#18029=EDGE_CURVE ( 'NONE', #11386, #706, #8216, .T. ) ;
#18046=ORIENTED_EDGE ( 'NONE', *, *, #15126, .F. ) ;
#18063=ADVANCED_FACE ( 'NONE', ( #3577 ), #10304, .T. ) ;
#18069=VERTEX_POINT ( 'NONE', #15144 ) ;
#18081=ORIENTED_EDGE ( 'NONE', *, *, #13428, .F. ) ;
#18108=ORIENTED_EDGE ( 'NONE', *, *, #10158, .T. ) ;
#18111=LINE ( 'NONE', #20013, #15735 ) ;
#18124=DIRECTION ( 'NONE',  ( 0.000000000000000000, -1.000000000000000000, 0.000000000000000000 ) ) ;
#18137=VECTOR ( 'NONE', #20950, 1000.000000000000000 ) ;
#18144=EDGE_CURVE ( 'NONE', #7658, #417, #16682, .T. ) ;
#18170=CARTESIAN_POINT ( 'NONE',  ( -176.9699209214867324, -126.9891397928655010, -72.64809332337415526 ) ) ;
#18183=ORIENTED_EDGE ( 'NONE', *, *, #2798, .T. ) ;
#18202=LINE ( 'NONE', #4755, #6125 ) ;
#18209=ORIENTED_EDGE ( 'NONE', *, *, #20245, .F. ) ;
#18221=ORIENTED_EDGE ( 'NONE', *, *, #12332, .T. ) ;
#18226=CIRCLE ( 'NONE', #14694, 10.00000000000000888 ) ;
#18247=PLANE ( 'NONE',  #16103 ) ;
#18259=DIRECTION ( 'NONE',  ( 0.000000000000000000, 0.000000000000000000, 1.000000000000000000 ) ) ;
#18290=CARTESIAN_POINT ( 'NONE',  ( -151.4692556286852891, -126.9891397928655010, 59.65701158161632378 ) ) ;
#18322=ADVANCED_FACE ( 'NONE', ( #478 ), #19109, .F. ) ;
#18336=ORIENTED_EDGE ( 'NONE', *, *, #9932, .F. ) ;
#18338=ORIENTED_EDGE ( 'NONE', *, *, #15126, .T. ) ;
#18379=CARTESIAN_POINT ( 'NONE',  ( -9.888205435155610346, 14.72870593739803624, -25.00000000000000000 ) ) ;
#18381=LINE ( 'NONE', #3282, #21627 ) ;
#18390=EDGE_CURVE ( 'NONE', #10043, #4009, #12475, .T. ) ;
#18399=EDGE_CURVE ( 'NONE', #12683, #18667, #14575, .T. ) ;
#18402=LINE ( 'NONE', #1535, #16072 ) ;
#18424=CARTESIAN_POINT ( 'NONE',  ( 147.8787791192428074, -136.9891397928655010, 59.65701158161630957 ) ) ;
#18433=CYLINDRICAL_SURFACE ( 'NONE', #21712, 10.00000000000003730 ) ;
#18449=EDGE_LOOP ( 'NONE', ( #7094, #6315, #5077, #12638, #20513, #14394, #16878, #5963, #3035 ) ) ;
#18451=VERTEX_POINT ( 'NONE', #4318 ) ;
#18461=CARTESIAN_POINT ( 'NONE',  ( 116.9721770337685740, 133.1239846058259388, -25.00000000000000000 ) ) ;
#18466=VECTOR ( 'NONE', #9055, 1000.000000000000000 ) ;
#18477=CARTESIAN_POINT ( 'NONE',  ( 121.4021762516569964, 137.5714195593754710, -35.00000000000000000 ) ) ;
#18479=DIRECTION ( 'NONE',  ( 0.000000000000000000, 0.000000000000000000, 1.000000000000000000 ) ) ;
#18482=CARTESIAN_POINT ( 'NONE',  ( 76.17254549292280785, -61.68114226949890622, 30.00000000000000000 ) ) ;
#18512=DIRECTION ( 'NONE',  ( -1.000000000000000000, -0.000000000000000000, -0.000000000000000000 ) ) ;
#18514=DIRECTION ( 'NONE',  ( -1.140132994654635861E-16, -0.000000000000000000, -1.000000000000000000 ) ) ;
#18529=VERTEX_POINT ( 'NONE', #11811 ) ;
#18540=EDGE_CURVE ( 'NONE', #8611, #15790, #18202, .T. ) ;
#18566=CARTESIAN_POINT ( 'NONE',  ( 126.8576204525573274, -126.9891397928655010, -17.64809332337413750 ) ) ;
#18571=FACE_OUTER_BOUND ( 'NONE', #16966, .T. ) ;
#18598=DIRECTION ( 'NONE',  ( 0.000000000000000000, -1.000000000000000000, 0.000000000000000000 ) ) ;
#18620=FACE_OUTER_BOUND ( 'NONE', #5004, .T. ) ;
#18629=CIRCLE ( 'NONE', #668, 10.00000000000003730 ) ;
#18638=VERTEX_POINT ( 'NONE', #10060 ) ;
#18653=CARTESIAN_POINT ( 'NONE',  ( 116.4417310231185780, -126.9891397928655010, 0.3429884183836981459 ) ) ;
#18667=VERTEX_POINT ( 'NONE', #17194 ) ;
#18674=AXIS2_PLACEMENT_3D ( 'NONE', #678, #7631, #1005 ) ;
#18688=EDGE_CURVE ( 'NONE', #10043, #16938, #19187, .T. ) ;
#18740=DIRECTION ( 'NONE',  ( 0.000000000000000000, 0.000000000000000000, 1.000000000000000000 ) ) ;
#18790=CARTESIAN_POINT ( 'NONE',  ( -130.4480969619997950, -126.9891397928655010, -72.64809332337412684 ) ) ;
#18825=EDGE_CURVE ( 'NONE', #9693, #9727, #10018, .T. ) ;
#18835=DIRECTION ( 'NONE',  ( 0.000000000000000000, 0.000000000000000000, 1.000000000000000000 ) ) ;
#18896=CARTESIAN_POINT ( 'NONE',  ( -176.9699209214867608, 72.84679049016736485, -35.00000000000000000 ) ) ;
#18897=ORIENTED_EDGE ( 'NONE', *, *, #7768, .T. ) ;
#18916=CARTESIAN_POINT ( 'NONE',  ( 76.17254549292280785, -61.68114226949890622, 20.00000000000000355 ) ) ;
#18926=AXIS2_PLACEMENT_3D ( 'NONE', #15146, #1707, #12266 ) ;
#18932=CARTESIAN_POINT ( 'NONE',  ( -130.4480969619997950, -136.9891397928655010, -72.64809332337412684 ) ) ;
#18933=EDGE_CURVE ( 'NONE', #15277, #12363, #1101, .T. ) ;
#18935=ORIENTED_EDGE ( 'NONE', *, *, #18825, .T. ) ;
#18938=CARTESIAN_POINT ( 'NONE',  ( -40.97538603781489996, -6.141859983696321912, -19.99999999999997513 ) ) ;
#18976=DIRECTION ( 'NONE',  ( 1.000000000000000000, 0.000000000000000000, 0.000000000000000000 ) ) ;
#18994=CARTESIAN_POINT ( 'NONE',  ( -151.4692556286852891, -126.9891397928655010, -64.65701158161634510 ) ) ;
#19001=CARTESIAN_POINT ( 'NONE',  ( -176.9699209214867892, -4.918956727831215833E-14, 30.00000000000000000 ) ) ;
#19008=LINE ( 'NONE', #5545, #11667 ) ;
#19015=ORIENTED_EDGE ( 'NONE', *, *, #12154, .T. ) ;
#19016=FACE_OUTER_BOUND ( 'NONE', #10714, .T. ) ;
#19017=ADVANCED_FACE ( 'NONE', ( #16738 ), #5650, .F. ) ;
#19022=CYLINDRICAL_SURFACE ( 'NONE', #13628, 7.500000000000000000 ) ;
#19027=CARTESIAN_POINT ( 'NONE',  ( 76.17254549292280785, -61.68114226949890622, -46.21320343559645494 ) ) ;
#19051=CARTESIAN_POINT ( 'NONE',  ( 116.4417310231185780, -136.9891397928655010, 49.65701158161629536 ) ) ;
#19062=CARTESIAN_POINT ( 'NONE',  ( 83.67254549292280785, -61.68114226949890622, 30.00000000000000000 ) ) ;
#19092=EDGE_LOOP ( 'NONE', ( #6902, #2984, #17775, #4528 ) ) ;
#19093=AXIS2_PLACEMENT_3D ( 'NONE', #10375, #17076, #5723 ) ;
#19095=CIRCLE ( 'NONE', #9590, 10.00000000000000888 ) ;
#19109=PLANE ( 'NONE',  #21283 ) ;
#19112=LINE ( 'NONE', #10525, #5199 ) ;
#19114=EDGE_LOOP ( 'NONE', ( #7697, #3099, #4199, #20325 ) ) ;
#19167=CARTESIAN_POINT ( 'NONE',  ( -130.4480969619998234, -136.9891397928655010, 67.64809332337415526 ) ) ;
#19175=ORIENTED_EDGE ( 'NONE', *, *, #18029, .F. ) ;
#19178=ADVANCED_FACE ( 'NONE', ( #8920, #9028, #10679, #12212, #10573 ), #13971, .T. ) ;
#19187=LINE ( 'NONE', #4086, #18466 ) ;
#19188=CYLINDRICAL_SURFACE ( 'NONE', #9446, 10.00000000000000888 ) ;
#19200=ORIENTED_EDGE ( 'NONE', *, *, #15281, .T. ) ;
#19228=ORIENTED_EDGE ( 'NONE', *, *, #6178, .T. ) ;
#19234=DIRECTION ( 'NONE',  ( -1.186952418100008983E-16, -0.000000000000000000, -1.000000000000000000 ) ) ;
#19235=LINE ( 'NONE', #8893, #14142 ) ;
#19236=AXIS2_PLACEMENT_3D ( 'NONE', #3353, #1702, #8431 ) ;
#19268=CARTESIAN_POINT ( 'NONE',  ( -120.0322075325610740, -126.9891397928655010, 30.00000000000000000 ) ) ;
#19278=FACE_OUTER_BOUND ( 'NONE', #4800, .T. ) ;
#19284=ORIENTED_EDGE ( 'NONE', *, *, #10557, .F. ) ;
#19292=LINE ( 'NONE', #14536, #18137 ) ;
#19310=EDGE_LOOP ( 'NONE', ( #11462, #10664 ) ) ;
#19333=CARTESIAN_POINT ( 'NONE',  ( 173.3794444120442506, -37.13255853780189852, 30.00000000000000000 ) ) ;
#19338=LINE ( 'NONE', #21004, #20842 ) ;
#19342=CARTESIAN_POINT ( 'NONE',  ( -47.86331837773882825, 0.000000000000000000, -19.99999999999997513 ) ) ;
#19345=EDGE_CURVE ( 'NONE', #11274, #16314, #15947, .T. ) ;
#19400=DIRECTION ( 'NONE',  ( -0.8302490056034133037, -0.5573926701119628069, 0.000000000000000000 ) ) ;
#19403=VERTEX_POINT ( 'NONE', #4369 ) ;
#19406=VERTEX_POINT ( 'NONE', #7486 ) ;
#19409=ORIENTED_EDGE ( 'NONE', *, *, #6927, .F. ) ;
#19413=EDGE_CURVE ( 'NONE', #40, #21314, #9570, .T. ) ;
#19427=CARTESIAN_POINT ( 'NONE',  ( 126.8576204525573274, -126.9891397928655010, -17.64809332337413750 ) ) ;
#19488=DIRECTION ( 'NONE',  ( 0.000000000000000000, 0.000000000000000000, 1.000000000000000000 ) ) ;
#19491=DIRECTION ( 'NONE',  ( -0.000000000000000000, -0.000000000000000000, 1.000000000000000000 ) ) ;
#19510=ORIENTED_EDGE ( 'NONE', *, *, #14991, .F. ) ;
#19519=ADVANCED_FACE ( 'NONE', ( #4268 ), #10787, .F. ) ;
#19521=ORIENTED_EDGE ( 'NONE', *, *, #3391, .T. ) ;
#19530=CARTESIAN_POINT ( 'NONE',  ( -120.0322075325610740, -136.9891397928655010, 30.00000000000000000 ) ) ;
#19532=ORIENTED_EDGE ( 'NONE', *, *, #18390, .F. ) ;
#19553=CARTESIAN_POINT ( 'NONE',  ( -176.9699209214867608, -126.9891397928655010, 30.00000000000000000 ) ) ;
#19563=EDGE_LOOP ( 'NONE', ( #12583, #16368, #20317, #27, #20997, #19570, #12880, #10423 ) ) ;
#19564=FACE_BOUND ( 'NONE', #15051, .T. ) ;
#19566=ADVANCED_FACE ( 'NONE', ( #14514, #12864, #19585 ), #16053, .F. ) ;
#19570=ORIENTED_EDGE ( 'NONE', *, *, #19577, .T. ) ;
#19575=VECTOR ( 'NONE', #5967, 1000.000000000000000 ) ;
#19577=EDGE_CURVE ( 'NONE', #5667, #735, #2507, .T. ) ;
#19582=CARTESIAN_POINT ( 'NONE',  ( 147.8787791192428074, -126.9891397928655010, 0.3429884183836981459 ) ) ;
#19585=FACE_OUTER_BOUND ( 'NONE', #3667, .T. ) ;
#19613=CARTESIAN_POINT ( 'NONE',  ( 173.3794444120442506, -126.9891397928655010, -17.64809332337413750 ) ) ;
#19635=EDGE_LOOP ( 'NONE', ( #17696, #7342, #5911, #13830 ) ) ;
#19648=DIRECTION ( 'NONE',  ( 1.186952418100008983E-16, 0.000000000000000000, 1.000000000000000000 ) ) ;
#19667=DIRECTION ( 'NONE',  ( 0.000000000000000000, -1.000000000000000000, 0.000000000000000000 ) ) ;
#19688=ORIENTED_EDGE ( 'NONE', *, *, #9067, .F. ) ;
#19692=EDGE_CURVE ( 'NONE', #14823, #15585, #11420, .T. ) ;
#19694=DIRECTION ( 'NONE',  ( 0.000000000000000000, 1.000000000000000000, 0.000000000000000000 ) ) ;
#19724=PLANE ( 'NONE',  #6199 ) ;
#19730=DIRECTION ( 'NONE',  ( 0.000000000000000000, -1.000000000000000000, 0.000000000000000000 ) ) ;
#19743=EDGE_LOOP ( 'NONE', ( #2872, #11323, #3485, #12882 ) ) ;
#19759=DIRECTION ( 'NONE',  ( -1.140132994654635861E-16, -0.000000000000000000, -1.000000000000000000 ) ) ;
#19770=VERTEX_POINT ( 'NONE', #13840 ) ;
#19775=ADVANCED_FACE ( 'NONE', ( #6918 ), #5146, .F. ) ;
#19777=AXIS2_PLACEMENT_3D ( 'NONE', #14302, #21260, #6139 ) ;
#19783=LINE ( 'NONE', #4676, #21053 ) ;
#19824=FACE_BOUND ( 'NONE', #19310, .T. ) ;
#19835=CARTESIAN_POINT ( 'NONE',  ( -176.9699209214867608, -126.9891397928655010, 67.64809332337415526 ) ) ;
#19836=CARTESIAN_POINT ( 'NONE',  ( -176.9699209214867324, -126.9891397928655010, -72.64809332337415526 ) ) ;
#19855=APPLICATION_CONTEXT ( 'automotive_design' ) ;
#19858=EDGE_CURVE ( 'NONE', #6015, #3147, #4035, .T. ) ;
#19865=EDGE_CURVE ( 'NONE', #18529, #4573, #11069, .T. ) ;
#19917=AXIS2_PLACEMENT_3D ( 'NONE', #9734, #8077, #19985 ) ;
#19942=FACE_OUTER_BOUND ( 'NONE', #19563, .T. ) ;
#19945=DIRECTION ( 'NONE',  ( 0.000000000000000000, 0.000000000000000000, 1.000000000000000000 ) ) ;
#19985=DIRECTION ( 'NONE',  ( 1.000000000000000000, 0.000000000000000000, 0.000000000000000000 ) ) ;
#20003=VECTOR ( 'NONE', #21237, 1000.000000000000227 ) ;
#20013=CARTESIAN_POINT ( 'NONE',  ( -130.4480969619997950, -126.9891397928655010, -72.64809332337412684 ) ) ;
#20024=ADVANCED_FACE ( 'NONE', ( #12045 ), #7206, .T. ) ;
#20027=DIRECTION ( 'NONE',  ( -1.000000000000000000, 0.000000000000000000, 0.000000000000000000 ) ) ;
#20044=DIRECTION ( 'NONE',  ( 1.000000000000000000, 0.000000000000000000, 0.000000000000000000 ) ) ;
#20051=CARTESIAN_POINT ( 'NONE',  ( 126.8576204525573274, -126.9891397928655010, 67.64809332337412684 ) ) ;
#20096=CARTESIAN_POINT ( 'NONE',  ( -176.9699209214867608, -136.9891397928655010, 30.00000000000000000 ) ) ;
#20103=ORIENTED_EDGE ( 'NONE', *, *, #21681, .F. ) ;
#20108=VERTEX_POINT ( 'NONE', #10514 ) ;
#20131=LINE ( 'NONE', #11734, #3805 ) ;
#20140=VECTOR ( 'NONE', #1768, 1000.000000000000000 ) ;
#20141=DIRECTION ( 'NONE',  ( 1.000000000000000000, 0.000000000000000000, 0.000000000000000000 ) ) ;
#20167=CARTESIAN_POINT ( 'NONE',  ( 121.4021762516569964, 137.5714195593754710, -35.00000000000000000 ) ) ;
#20178=CARTESIAN_POINT ( 'NONE',  ( 116.4417310231185780, -126.9891397928655010, 19.99999999999999645 ) ) ;
#20180=DIRECTION ( 'NONE',  ( 0.000000000000000000, -1.000000000000000000, 0.000000000000000000 ) ) ;
#20185=ORIENTED_EDGE ( 'NONE', *, *, #16291, .F. ) ;
#20193=VERTEX_POINT ( 'NONE', #6375 ) ;
#20227=CARTESIAN_POINT ( 'NONE',  ( 132.3486983259487886, 110.2203079035327420, -25.00000000000000000 ) ) ;
#20236=VECTOR ( 'NONE', #2856, 1000.000000000000000 ) ;
#20240=DIRECTION ( 'NONE',  ( -0.000000000000000000, -0.000000000000000000, 1.000000000000000000 ) ) ;
#20245=EDGE_CURVE ( 'NONE', #2574, #6176, #6684, .T. ) ;
#20253=LINE ( 'NONE', #2161, #2994 ) ;
#20267=EDGE_LOOP ( 'NONE', ( #12716, #12421, #5722, #17750 ) ) ;
#20269=PLANE ( 'NONE',  #11173 ) ;
#20278=EDGE_CURVE ( 'NONE', #4745, #13613, #18629, .T. ) ;
#20306=CARTESIAN_POINT ( 'NONE',  ( -151.4692556286852891, -136.9891397928655010, -54.65701158161630246 ) ) ;
#20317=ORIENTED_EDGE ( 'NONE', *, *, #7587, .F. ) ;
#20319=DIRECTION ( 'NONE',  ( 0.000000000000000000, -0.000000000000000000, -1.000000000000000000 ) ) ;
#20322=VERTEX_POINT ( 'NONE', #3183 ) ;
#20325=ORIENTED_EDGE ( 'NONE', *, *, #11916, .T. ) ;
#20352=ORIENTED_EDGE ( 'NONE', *, *, #5164, .T. ) ;
#20362=DIRECTION ( 'NONE',  ( 0.000000000000000000, 0.000000000000000000, -1.000000000000000000 ) ) ;
#20383=LINE ( 'NONE', #13542, #8328 ) ;
#20417=CARTESIAN_POINT ( 'NONE',  ( -176.9699209214867608, -136.9891397928655010, 67.64809332337415526 ) ) ;
#20424=PRODUCT_DEFINITION_FORMATION_WITH_SPECIFIED_SOURCE ( 'ANY', '', #13296, .NOT_KNOWN. ) ;
#20484=EDGE_LOOP ( 'NONE', ( #8256, #10531, #21132, #21404 ) ) ;
#20496=AXIS2_PLACEMENT_3D ( 'NONE', #11503, #8435, #11945 ) ;
#20503=AXIS2_PLACEMENT_3D ( 'NONE', #18379, #10010, #19400 ) ;
#20512=EDGE_CURVE ( 'NONE', #2203, #17644, #9131, .T. ) ;
#20513=ORIENTED_EDGE ( 'NONE', *, *, #6806, .T. ) ;
#20520=DIRECTION ( 'NONE',  ( 0.000000000000000000, -1.000000000000000000, 0.000000000000000000 ) ) ;
#20537=ORIENTED_EDGE ( 'NONE', *, *, #18540, .T. ) ;
#20539=ORIENTED_EDGE ( 'NONE', *, *, #20679, .F. ) ;
#20554=DIRECTION ( 'NONE',  ( -0.000000000000000000, -1.000000000000000000, -0.000000000000000000 ) ) ;
#20570=LINE ( 'NONE', #1729, #10451 ) ;
#20571=VECTOR ( 'NONE', #6134, 1000.000000000000000 ) ;
#20574=DIRECTION ( 'NONE',  ( 0.000000000000000000, 0.000000000000000000, -1.000000000000000000 ) ) ;
#20611=ADVANCED_FACE ( 'NONE', ( #98 ), #16941, .F. ) ;
#20640=DIRECTION ( 'NONE',  ( 0.8654262854811264338, 0.000000000000000000, -0.5010362705417042983 ) ) ;
#20648=DIRECTION ( 'NONE',  ( -0.000000000000000000, -0.000000000000000000, -1.000000000000000000 ) ) ;
#20679=EDGE_CURVE ( 'NONE', #11465, #9722, #15111, .T. ) ;
#20690=CIRCLE ( 'NONE', #3789, 7.500000000000007105 ) ;
#20708=FACE_OUTER_BOUND ( 'NONE', #5006, .T. ) ;
#20722=VERTEX_POINT ( 'NONE', #15939 ) ;
#20725=VERTEX_POINT ( 'NONE', #18938 ) ;
#20758=DIRECTION ( 'NONE',  ( -1.233581138472395521E-15, 0.000000000000000000, 1.000000000000000000 ) ) ;
#20765=EDGE_LOOP ( 'NONE', ( #19688, #13952 ) ) ;
#20781=EDGE_CURVE ( 'NONE', #17291, #4877, #8805, .T. ) ;
#20782=DIRECTION ( 'NONE',  ( 0.000000000000000000, -1.000000000000000000, 0.000000000000000000 ) ) ;
#20786=LINE ( 'NONE', #19553, #9776 ) ;
#20803=EDGE_CURVE ( 'NONE', #7232, #10397, #21572, .T. ) ;
#20805=ORIENTED_EDGE ( 'NONE', *, *, #1282, .T. ) ;
#20830=ORIENTED_EDGE ( 'NONE', *, *, #20803, .T. ) ;
#20842=VECTOR ( 'NONE', #4238, 1000.000000000000000 ) ;
#20853=AXIS2_PLACEMENT_3D ( 'NONE', #1304, #9694, #1194 ) ;
#20879=ORIENTED_EDGE ( 'NONE', *, *, #4244, .T. ) ;
#20907=EDGE_CURVE ( 'NONE', #4859, #18638, #11302, .T. ) ;
#20940=COLOUR_RGB ( '', 0.66274510, 0.83137255, 0.94901961) ;
#20950=DIRECTION ( 'NONE',  ( 0.000000000000000000, -1.000000000000000000, 0.000000000000000000 ) ) ;
#20953=DIRECTION ( 'NONE',  ( 1.000000000000000000, 0.000000000000000000, 0.000000000000000000 ) ) ;
#20957=AXIS2_PLACEMENT_3D ( 'NONE', #2841, #14417, #1192 ) ;
#20979=DIRECTION ( 'NONE',  ( -2.779543948608941985E-16, 1.000000000000000000, 0.000000000000000000 ) ) ;
#20992=CYLINDRICAL_SURFACE ( 'NONE', #2527, 10.00000000000000888 ) ;
#20997=ORIENTED_EDGE ( 'NONE', *, *, #12332, .F. ) ;
#21004=CARTESIAN_POINT ( 'NONE',  ( -176.9699209214867608, 160.7104996726487514, -35.00000000000000000 ) ) ;
#21009=DIRECTION ( 'NONE',  ( 0.000000000000000000, 1.000000000000000000, -0.000000000000000000 ) ) ;
#21027=ORIENTED_EDGE ( 'NONE', *, *, #3684, .T. ) ;
#21053=VECTOR ( 'NONE', #9762, 1000.000000000000000 ) ;
#21081=ADVANCED_FACE ( 'NONE', ( #17804 ), #9782, .T. ) ;
#21083=ORIENTED_EDGE ( 'NONE', *, *, #11834, .F. ) ;
#21094=CARTESIAN_POINT ( 'NONE',  ( -151.4692556286852891, -136.9891397928655010, 49.65701158161630957 ) ) ;
#21096=EDGE_LOOP ( 'NONE', ( #17309, #1279, #4713, #21083, #2873 ) ) ;
#21107=DIRECTION ( 'NONE',  ( -0.000000000000000000, -0.000000000000000000, -1.000000000000000000 ) ) ;
#21112=CARTESIAN_POINT ( 'NONE',  ( -32.30114424549768870, -19.06233958201669410, -19.99999999999997513 ) ) ;
#21115=FACE_OUTER_BOUND ( 'NONE', #11029, .T. ) ;
#21126=EDGE_CURVE ( 'NONE', #12769, #9727, #15280, .T. ) ;
#21132=ORIENTED_EDGE ( 'NONE', *, *, #17075, .T. ) ;
#21215=ORIENTED_EDGE ( 'NONE', *, *, #6493, .T. ) ;
#21229=ADVANCED_FACE ( 'NONE', ( #9889, #3495 ), #16588, .T. ) ;
#21235=DIRECTION ( 'NONE',  ( 0.000000000000000000, -1.000000000000000000, 0.000000000000000000 ) ) ;
#21237=DIRECTION ( 'NONE',  ( -0.5010362705417047424, 0.000000000000000000, -0.8654262854811261008 ) ) ;
#21244=ORIENTED_EDGE ( 'NONE', *, *, #13822, .F. ) ;
#21255=CARTESIAN_POINT ( 'NONE',  ( 147.8787791192428074, -126.9891397928655010, -9.657011581616311346 ) ) ;
#21260=DIRECTION ( 'NONE',  ( 1.000000000000000000, 0.000000000000000000, -0.000000000000000000 ) ) ;
#21264=CARTESIAN_POINT ( 'NONE',  ( 173.3794444120442506, -126.9891397928655010, 67.64809332337412684 ) ) ;
#21271=ADVANCED_FACE ( 'NONE', ( #1507 ), #1612, .F. ) ;
#21283=AXIS2_PLACEMENT_3D ( 'NONE', #12151, #14024, #20758 ) ;
#21289=MECHANICAL_DESIGN_GEOMETRIC_PRESENTATION_REPRESENTATION('',(#8969),#14280);
#21307=LINE ( 'NONE', #14787, #7319 ) ;
#21314=VERTEX_POINT ( 'NONE', #8994 ) ;
#21315=LINE ( 'NONE', #11269, #13243 ) ;
#21360=CIRCLE ( 'NONE', #4110, 15.56217413224114310 ) ;
#21368=CARTESIAN_POINT ( 'NONE',  ( 147.8787791192428074, -136.9891397928655010, 0.3429884183836981459 ) ) ;
#21370=EDGE_CURVE ( 'NONE', #17801, #12681, #13728, .T. ) ;
#21404=ORIENTED_EDGE ( 'NONE', *, *, #1668, .F. ) ;
#21407=VECTOR ( 'NONE', #4486, 1000.000000000000000 ) ;
#21426=ORIENTED_EDGE ( 'NONE', *, *, #1282, .F. ) ;
#21460=AXIS2_PLACEMENT_3D ( 'NONE', #13408, #8236, #20141 ) ;
#21486=ORIENTED_EDGE ( 'NONE', *, *, #12200, .T. ) ;
#21498=EDGE_CURVE ( 'NONE', #17801, #14823, #7131, .T. ) ;
#21548=DIRECTION ( 'NONE',  ( 0.000000000000000000, 1.000000000000000000, 0.000000000000000000 ) ) ;
#21569=ORIENTED_EDGE ( 'NONE', *, *, #7039, .T. ) ;
#21572=LINE ( 'NONE', #6352, #4906 ) ;
#21611=DIRECTION ( 'NONE',  ( -1.000000000000000000, 0.000000000000000000, 1.186952418100008737E-16 ) ) ;
#21627=VECTOR ( 'NONE', #16717, 1000.000000000000000 ) ;
#21629=EDGE_LOOP ( 'NONE', ( #2331, #12142, #15191, #10955 ) ) ;
#21635=VECTOR ( 'NONE', #858, 1000.000000000000000 ) ;
#21651=LINE ( 'NONE', #4884, #8872 ) ;
#21652=AXIS2_PLACEMENT_3D ( 'NONE', #16165, #2404, #2611 ) ;
#21665=CARTESIAN_POINT ( 'NONE',  ( 173.3794444120442506, -126.9891397928655010, 30.00000000000000000 ) ) ;
#21681=EDGE_CURVE ( 'NONE', #4525, #19770, #14479, .T. ) ;
#21705=VERTEX_POINT ( 'NONE', #4674 ) ;
#21712=AXIS2_PLACEMENT_3D ( 'NONE', #10061, #5409, #10277 ) ;
#21733=ORIENTED_EDGE ( 'NONE', *, *, #3276, .T. ) ;
#21749=VERTEX_POINT ( 'NONE', #4447 ) ;
#21766=VECTOR ( 'NONE', #5014, 1000.000000000000000 ) ;
#21772=LINE ( 'NONE', #6677, #21766 ) ;
#21783=DIRECTION ( 'NONE',  ( 0.000000000000000000, 0.000000000000000000, 1.000000000000000000 ) ) ;
#21793=DIRECTION ( 'NONE',  ( 0.000000000000000000, 1.000000000000000000, -0.000000000000000000 ) ) ;
ENDSEC;
END-ISO-10303-21;
